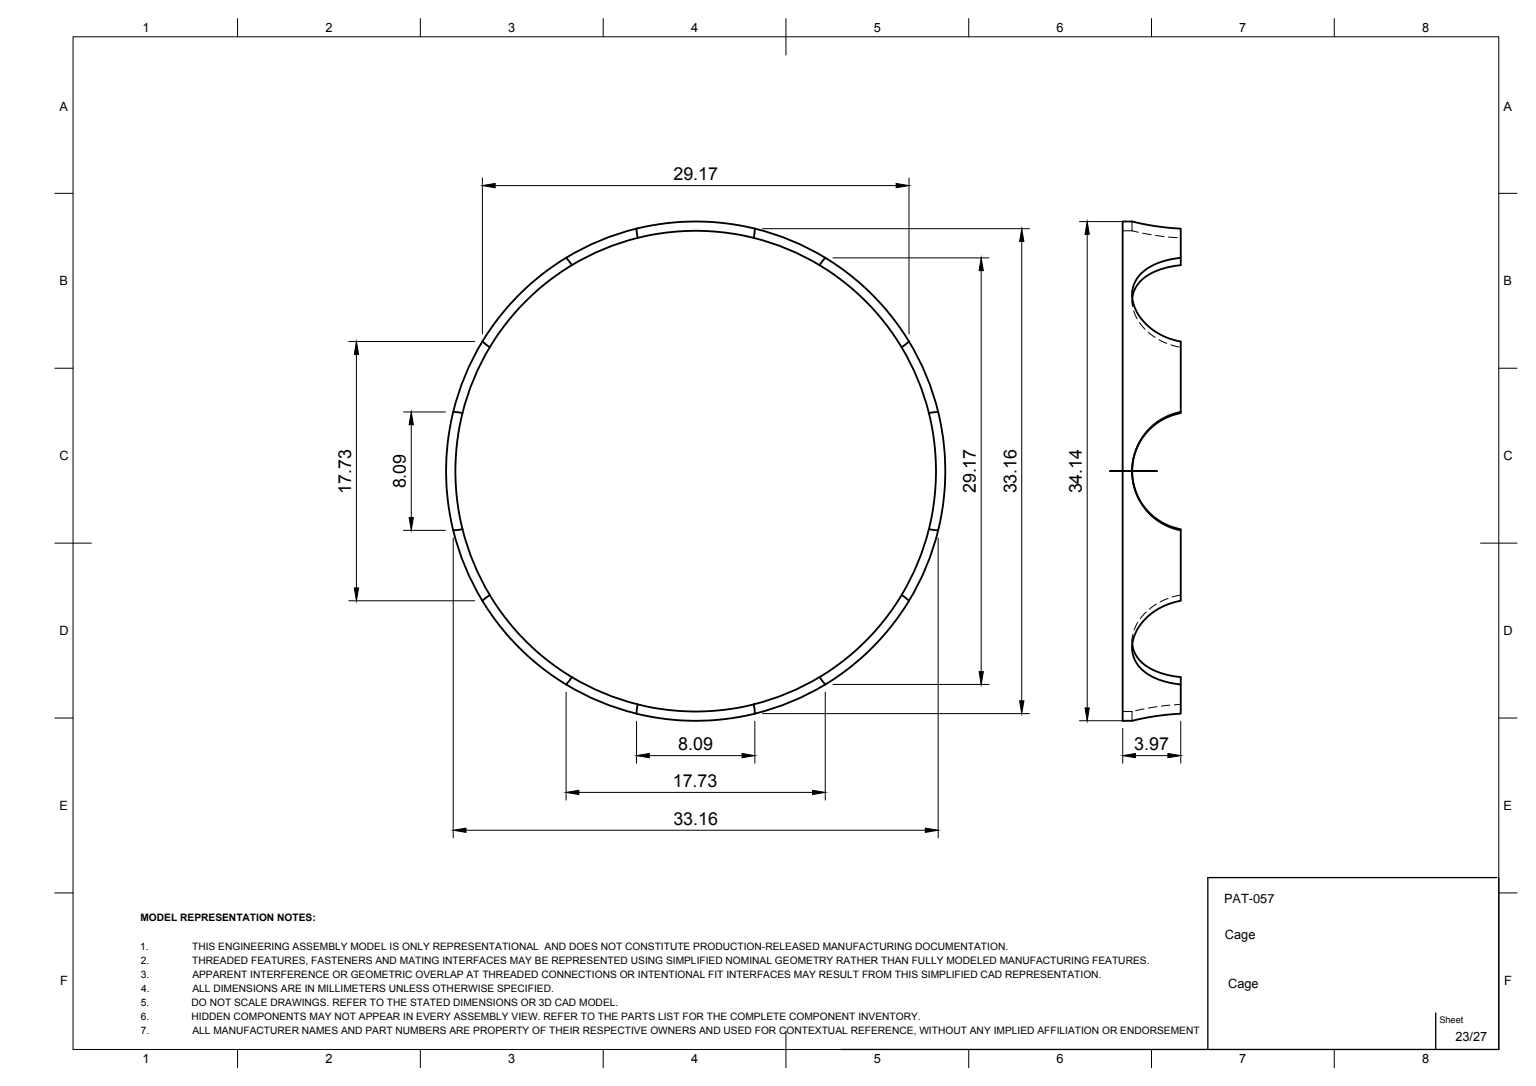
ISO-10303-21;
HEADER;
/* Generated by software containing ST-Developer
 * from STEP Tools, Inc. (www.steptools.com) 
 */

FILE_DESCRIPTION(
/* description */ ('Bearing-mounted hook block'),
/* implementation_level */ '2;1');

FILE_NAME(
/* name */ 'Cage.step',
/* time_stamp */ '2026-10-28T22:30:11-07:00',
/* author */ (''),
/* organization */ (''),
/* preprocessor_version */ 'ST-DEVELOPER v20.2',
/* originating_system */ 'Autodesk Translation Framework v15.17.0.0',
/* authorisation */ '');

FILE_SCHEMA (('AUTOMOTIVE_DESIGN { 1 0 10303 214 3 1 1 }'));
ENDSEC;

DATA;
#10=MECHANICAL_DESIGN_GEOMETRIC_PRESENTATION_REPRESENTATION('',(#347),#7609);
#11=B_SPLINE_CURVE_WITH_KNOTS('',3,(#6806,#6807,#6808,#6809,#6810,#6811,
#6812,#6813,#6814,#6815,#6816,#6817,#6818,#6819,#6820,#6821,#6822,#6823,
#6824,#6825,#6826,#6827),.UNSPECIFIED.,.F.,.F.,(4,2,2,2,2,2,2,2,2,2,4),
(0.0789094028588958,0.210573405340968,0.315860108011452,0.421146810681936,
0.522142632548711,0.623138454415485,0.72413427628226,0.825130098149035,
0.930416800819519,1.03570350349,1.16736750597208),.UNSPECIFIED.);
#12=B_SPLINE_CURVE_WITH_KNOTS('',3,(#6831,#6832,#6833,#6834,#6835,#6836,
#6837,#6838,#6839,#6840,#6841,#6842,#6843,#6844,#6845,#6846,#6847,#6848,
#6849,#6850,#6851,#6852),.UNSPECIFIED.,.F.,.F.,(4,2,2,2,2,2,2,2,2,2,4),
(0.0774793363974613,0.142088896491891,0.284177792983782,0.411119756996526,
0.514392970548519,0.617666184100513,0.720939397652506,0.8242126112045,0.951154575217244,
1.09324347170913,1.15785303180356),.UNSPECIFIED.);
#13=B_SPLINE_CURVE_WITH_KNOTS('',3,(#6858,#6859,#6860,#6861,#6862,#6863,
#6864,#6865,#6866,#6867,#6868,#6869,#6870,#6871,#6872,#6873,#6874,#6875,
#6876,#6877,#6878,#6879),.UNSPECIFIED.,.F.,.F.,(4,2,2,2,2,2,2,2,2,2,4),
(0.0774793363974613,0.142088896491891,0.284177792983782,0.411119756996525,
0.514392970548519,0.617666184100513,0.720939397652506,0.8242126112045,0.951154575217243,
1.09324347170913,1.15785303180356),.UNSPECIFIED.);
#14=B_SPLINE_CURVE_WITH_KNOTS('',3,(#6883,#6884,#6885,#6886,#6887,#6888,
#6889,#6890,#6891,#6892,#6893,#6894,#6895,#6896,#6897,#6898,#6899,#6900,
#6901,#6902,#6903,#6904),.UNSPECIFIED.,.F.,.F.,(4,2,2,2,2,2,2,2,2,2,4),
(0.0774793363974614,0.142088896491891,0.284177792983781,0.411119756996525,
0.514392970548519,0.617666184100512,0.720939397652506,0.824212611204499,
0.951154575217243,1.09324347170913,1.15785303180356),.UNSPECIFIED.);
#15=B_SPLINE_CURVE_WITH_KNOTS('',3,(#6908,#6909,#6910,#6911,#6912,#6913,
#6914,#6915,#6916,#6917,#6918,#6919),.UNSPECIFIED.,.F.,.F.,(4,2,2,2,2,4),
(0.0774793363974613,0.142088896491891,0.284177792983781,0.411119756996525,
0.514392970548519,0.617666184100512),.UNSPECIFIED.);
#16=B_SPLINE_CURVE_WITH_KNOTS('',3,(#6924,#6925,#6926,#6927,#6928,#6929,
#6930,#6931,#6932,#6933,#6934,#6935),.UNSPECIFIED.,.F.,.F.,(4,2,2,2,2,4),
(0.617666184100512,0.720939397652506,0.824212611204499,0.951154575217243,
1.09324347170913,1.15785303180356),.UNSPECIFIED.);
#17=B_SPLINE_CURVE_WITH_KNOTS('',3,(#6939,#6940,#6941,#6942,#6943,#6944,
#6945,#6946,#6947,#6948,#6949,#6950,#6951,#6952,#6953,#6954,#6955,#6956,
#6957,#6958,#6959,#6960),.UNSPECIFIED.,.F.,.F.,(4,2,2,2,2,2,2,2,2,2,4),
(0.0774793363974613,0.142088896491891,0.284177792983782,0.411119756996526,
0.514392970548519,0.617666184100513,0.720939397652507,0.8242126112045,0.951154575217245,
1.09324347170914,1.15785303180356),.UNSPECIFIED.);
#18=B_SPLINE_CURVE_WITH_KNOTS('',3,(#6964,#6965,#6966,#6967,#6968,#6969,
#6970,#6971,#6972,#6973,#6974,#6975,#6976,#6977,#6978,#6979,#6980,#6981,
#6982,#6983,#6984,#6985),.UNSPECIFIED.,.F.,.F.,(4,2,2,2,2,2,2,2,2,2,4),
(0.0774793363974613,0.142088896491891,0.284177792983782,0.411119756996526,
0.514392970548519,0.617666184100513,0.720939397652506,0.824212611204499,
0.951154575217243,1.09324347170913,1.15785303180356),.UNSPECIFIED.);
#19=B_SPLINE_CURVE_WITH_KNOTS('',3,(#6989,#6990,#6991,#6992,#6993,#6994,
#6995,#6996,#6997,#6998,#6999,#7000,#7001,#7002,#7003,#7004,#7005,#7006,
#7007,#7008,#7009,#7010),.UNSPECIFIED.,.F.,.F.,(4,2,2,2,2,2,2,2,2,2,4),
(0.0774793363974613,0.142088896491891,0.284177792983782,0.411119756996526,
0.514392970548519,0.617666184100513,0.720939397652506,0.8242126112045,0.951154575217244,
1.09324347170913,1.15785303180356),.UNSPECIFIED.);
#20=B_SPLINE_CURVE_WITH_KNOTS('',3,(#7014,#7015,#7016,#7017,#7018,#7019,
#7020,#7021,#7022,#7023,#7024,#7025,#7026,#7027,#7028,#7029,#7030,#7031,
#7032,#7033,#7034,#7035),.UNSPECIFIED.,.F.,.F.,(4,2,2,2,2,2,2,2,2,2,4),
(0.0774793363974613,0.142088896491891,0.284177792983782,0.411119756996526,
0.514392970548519,0.617666184100513,0.720939397652506,0.8242126112045,0.951154575217243,
1.09324347170913,1.15785303180356),.UNSPECIFIED.);
#21=B_SPLINE_CURVE_WITH_KNOTS('',3,(#7043,#7044,#7045,#7046,#7047,#7048,
#7049,#7050,#7051,#7052,#7053,#7054,#7055,#7056,#7057,#7058,#7059,#7060,
#7061,#7062,#7063,#7064),.UNSPECIFIED.,.F.,.F.,(4,2,2,2,2,2,2,2,2,2,4),
(0.0789094028588958,0.210573405340968,0.315860108011452,0.421146810681936,
0.522142632548711,0.623138454415485,0.72413427628226,0.825130098149035,
0.930416800819519,1.03570350349,1.16736750597208),.UNSPECIFIED.);
#22=B_SPLINE_CURVE_WITH_KNOTS('',3,(#7072,#7073,#7074,#7075,#7076,#7077,
#7078,#7079,#7080,#7081,#7082,#7083,#7084,#7085,#7086,#7087,#7088,#7089,
#7090,#7091,#7092,#7093),.UNSPECIFIED.,.F.,.F.,(4,2,2,2,2,2,2,2,2,2,4),
(0.0789094028588958,0.210573405340969,0.315860108011453,0.421146810681937,
0.522142632548712,0.623138454415486,0.724134276282261,0.825130098149035,
0.930416800819519,1.03570350349,1.16736750597208),.UNSPECIFIED.);
#23=B_SPLINE_CURVE_WITH_KNOTS('',3,(#7102,#7103,#7104,#7105,#7106,#7107,
#7108,#7109,#7110,#7111,#7112,#7113),.UNSPECIFIED.,.F.,.F.,(4,2,2,2,2,4),
(0.0789094028588958,0.210573405340968,0.315860108011452,0.421146810681937,
0.522142632548711,0.623138454415486),.UNSPECIFIED.);
#24=B_SPLINE_CURVE_WITH_KNOTS('',3,(#7115,#7116,#7117,#7118,#7119,#7120,
#7121,#7122,#7123,#7124,#7125,#7126),.UNSPECIFIED.,.F.,.F.,(4,2,2,2,2,4),
(0.623138454415486,0.72413427628226,0.825130098149035,0.930416800819519,
1.03570350349,1.16736750597208),.UNSPECIFIED.);
#25=B_SPLINE_CURVE_WITH_KNOTS('',3,(#7133,#7134,#7135,#7136,#7137,#7138,
#7139,#7140,#7141,#7142,#7143,#7144,#7145,#7146,#7147,#7148,#7149,#7150,
#7151,#7152,#7153,#7154),.UNSPECIFIED.,.F.,.F.,(4,2,2,2,2,2,2,2,2,2,4),
(0.0789094028588958,0.210573405340968,0.315860108011452,0.421146810681936,
0.522142632548711,0.623138454415486,0.72413427628226,0.825130098149035,
0.930416800819519,1.03570350349,1.16736750597208),.UNSPECIFIED.);
#26=B_SPLINE_CURVE_WITH_KNOTS('',3,(#7162,#7163,#7164,#7165,#7166,#7167,
#7168,#7169,#7170,#7171,#7172,#7173,#7174,#7175,#7176,#7177,#7178,#7179,
#7180,#7181,#7182,#7183),.UNSPECIFIED.,.F.,.F.,(4,2,2,2,2,2,2,2,2,2,4),
(0.0789094028588957,0.210573405340968,0.315860108011452,0.421146810681936,
0.522142632548711,0.623138454415485,0.72413427628226,0.825130098149035,
0.930416800819519,1.03570350349,1.16736750597207),.UNSPECIFIED.);
#27=B_SPLINE_CURVE_WITH_KNOTS('',3,(#7191,#7192,#7193,#7194,#7195,#7196,
#7197,#7198,#7199,#7200,#7201,#7202,#7203,#7204,#7205,#7206,#7207,#7208,
#7209,#7210,#7211,#7212),.UNSPECIFIED.,.F.,.F.,(4,2,2,2,2,2,2,2,2,2,4),
(0.0789094028588958,0.210573405340968,0.315860108011452,0.421146810681936,
0.522142632548711,0.623138454415486,0.72413427628226,0.825130098149035,
0.930416800819519,1.03570350349,1.16736750597208),.UNSPECIFIED.);
#28=B_SPLINE_CURVE_WITH_KNOTS('',3,(#7221,#7222,#7223,#7224,#7225,#7226,
#7227,#7228,#7229,#7230,#7231,#7232,#7233,#7234,#7235,#7236,#7237,#7238,
#7239,#7240,#7241,#7242),.UNSPECIFIED.,.F.,.F.,(4,2,2,2,2,2,2,2,2,2,4),
(0.0789094028588958,0.210573405340968,0.315860108011452,0.421146810681936,
0.522142632548711,0.623138454415485,0.72413427628226,0.825130098149035,
0.930416800819519,1.03570350349,1.16736750597208),.UNSPECIFIED.);
#37=SPHERICAL_SURFACE('',#4562,0.412776);
#38=SPHERICAL_SURFACE('',#4578,0.412776);
#39=SPHERICAL_SURFACE('',#4583,0.412776);
#40=SPHERICAL_SURFACE('',#4588,0.412776);
#41=SPHERICAL_SURFACE('',#4593,0.412776);
#42=SPHERICAL_SURFACE('',#4598,0.412776);
#43=SPHERICAL_SURFACE('',#4603,0.412776);
#44=SPHERICAL_SURFACE('',#4611,0.412776);
#292=SHAPE_REPRESENTATION_RELATIONSHIP('SRR','None',#7741,#316);
#316=ADVANCED_BREP_SHAPE_REPRESENTATION('',(#377),#7601);
#347=STYLED_ITEM('',(#7931),#377);
#377=MANIFOLD_SOLID_BREP('Continuous crown cage',#3945);
#535=LINE('',#6921,#765);
#536=LINE('',#7217,#766);
#765=VECTOR('',#5608,1.706752);
#766=VECTOR('',#5685,1.643248);
#898=CYLINDRICAL_SURFACE('',#4565,1.706752);
#899=CYLINDRICAL_SURFACE('',#4605,1.643248);
#978=FACE_BOUND('',#1466,.T.);
#1155=FACE_OUTER_BOUND('',#1448,.T.);
#1156=FACE_OUTER_BOUND('',#1449,.T.);
#1157=FACE_OUTER_BOUND('',#1450,.T.);
#1158=FACE_OUTER_BOUND('',#1451,.T.);
#1159=FACE_OUTER_BOUND('',#1452,.T.);
#1160=FACE_OUTER_BOUND('',#1453,.T.);
#1161=FACE_OUTER_BOUND('',#1454,.T.);
#1162=FACE_OUTER_BOUND('',#1455,.T.);
#1163=FACE_OUTER_BOUND('',#1456,.T.);
#1164=FACE_OUTER_BOUND('',#1457,.T.);
#1165=FACE_OUTER_BOUND('',#1458,.T.);
#1166=FACE_OUTER_BOUND('',#1459,.T.);
#1167=FACE_OUTER_BOUND('',#1460,.T.);
#1168=FACE_OUTER_BOUND('',#1461,.T.);
#1169=FACE_OUTER_BOUND('',#1462,.T.);
#1170=FACE_OUTER_BOUND('',#1463,.T.);
#1171=FACE_OUTER_BOUND('',#1464,.T.);
#1172=FACE_OUTER_BOUND('',#1465,.T.);
#1173=FACE_OUTER_BOUND('',#1467,.T.);
#1448=EDGE_LOOP('',(#3204,#3205,#3206,#3207));
#1449=EDGE_LOOP('',(#3208,#3209,#3210,#3211,#3212,#3213,#3214,#3215,#3216,
#3217,#3218,#3219,#3220,#3221,#3222,#3223,#3224,#3225,#3226,#3227));
#1450=EDGE_LOOP('',(#3228,#3229,#3230,#3231));
#1451=EDGE_LOOP('',(#3232,#3233,#3234,#3235));
#1452=EDGE_LOOP('',(#3236,#3237,#3238,#3239));
#1453=EDGE_LOOP('',(#3240,#3241,#3242,#3243));
#1454=EDGE_LOOP('',(#3244,#3245,#3246,#3247));
#1455=EDGE_LOOP('',(#3248,#3249,#3250,#3251,#3252,#3253));
#1456=EDGE_LOOP('',(#3254,#3255,#3256,#3257));
#1457=EDGE_LOOP('',(#3258,#3259,#3260,#3261));
#1458=EDGE_LOOP('',(#3262,#3263,#3264,#3265));
#1459=EDGE_LOOP('',(#3266,#3267,#3268,#3269));
#1460=EDGE_LOOP('',(#3270,#3271,#3272,#3273));
#1461=EDGE_LOOP('',(#3274,#3275,#3276,#3277));
#1462=EDGE_LOOP('',(#3278,#3279,#3280,#3281,#3282,#3283,#3284,#3285,#3286,
#3287,#3288,#3289,#3290,#3291,#3292,#3293,#3294,#3295,#3296,#3297));
#1463=EDGE_LOOP('',(#3298,#3299,#3300,#3301));
#1464=EDGE_LOOP('',(#3302,#3303,#3304,#3305));
#1465=EDGE_LOOP('',(#3306));
#1466=EDGE_LOOP('',(#3307));
#1467=EDGE_LOOP('',(#3308,#3309,#3310,#3311));
#1697=CIRCLE('',#4563,0.405071403305639);
#1698=CIRCLE('',#4564,0.405071403305639);
#1699=CIRCLE('',#4566,1.706752);
#1700=CIRCLE('',#4567,1.706752);
#1701=CIRCLE('',#4568,1.706752);
#1702=CIRCLE('',#4569,1.706752);
#1703=CIRCLE('',#4570,1.706752);
#1704=CIRCLE('',#4571,1.706752);
#1705=CIRCLE('',#4572,1.706752);
#1706=CIRCLE('',#4573,1.706752);
#1707=CIRCLE('',#4574,1.706752);
#1708=CIRCLE('',#4576,1.643248);
#1709=CIRCLE('',#4577,0.405071403305639);
#1710=CIRCLE('',#4579,0.405071403305639);
#1711=CIRCLE('',#4581,1.643248);
#1712=CIRCLE('',#4582,0.405071403305639);
#1713=CIRCLE('',#4584,0.405071403305639);
#1714=CIRCLE('',#4586,1.643248);
#1715=CIRCLE('',#4587,0.405071403305639);
#1716=CIRCLE('',#4589,0.405071403305639);
#1717=CIRCLE('',#4591,1.643248);
#1718=CIRCLE('',#4592,0.405071403305639);
#1719=CIRCLE('',#4594,0.405071403305639);
#1720=CIRCLE('',#4596,1.643248);
#1721=CIRCLE('',#4597,0.405071403305639);
#1722=CIRCLE('',#4599,0.405071403305639);
#1723=CIRCLE('',#4601,1.643248);
#1724=CIRCLE('',#4602,0.405071403305639);
#1725=CIRCLE('',#4604,0.405071403305639);
#1726=CIRCLE('',#4606,1.643248);
#1727=CIRCLE('',#4607,1.643248);
#1728=CIRCLE('',#4608,1.643248);
#1729=CIRCLE('',#4610,0.405071403305639);
#1730=CIRCLE('',#4612,0.405071403305639);
#1988=VERTEX_POINT('',#6804);
#1989=VERTEX_POINT('',#6805);
#1990=VERTEX_POINT('',#6828);
#1991=VERTEX_POINT('',#6830);
#1992=VERTEX_POINT('',#6855);
#1993=VERTEX_POINT('',#6857);
#1994=VERTEX_POINT('',#6880);
#1995=VERTEX_POINT('',#6882);
#1996=VERTEX_POINT('',#6905);
#1997=VERTEX_POINT('',#6907);
#1998=VERTEX_POINT('',#6920);
#1999=VERTEX_POINT('',#6923);
#2000=VERTEX_POINT('',#6936);
#2001=VERTEX_POINT('',#6938);
#2002=VERTEX_POINT('',#6961);
#2003=VERTEX_POINT('',#6963);
#2004=VERTEX_POINT('',#6986);
#2005=VERTEX_POINT('',#6988);
#2006=VERTEX_POINT('',#7011);
#2007=VERTEX_POINT('',#7013);
#2008=VERTEX_POINT('',#7038);
#2009=VERTEX_POINT('',#7042);
#2010=VERTEX_POINT('',#7067);
#2011=VERTEX_POINT('',#7071);
#2012=VERTEX_POINT('',#7096);
#2013=VERTEX_POINT('',#7100);
#2014=VERTEX_POINT('',#7101);
#2015=VERTEX_POINT('',#7128);
#2016=VERTEX_POINT('',#7132);
#2017=VERTEX_POINT('',#7157);
#2018=VERTEX_POINT('',#7161);
#2019=VERTEX_POINT('',#7186);
#2020=VERTEX_POINT('',#7190);
#2021=VERTEX_POINT('',#7215);
#2022=VERTEX_POINT('',#7218);
#2023=VERTEX_POINT('',#7220);
#2412=EDGE_CURVE('',#1988,#1989,#11,.T.);
#2413=EDGE_CURVE('',#1990,#1988,#1697,.T.);
#2414=EDGE_CURVE('',#1991,#1990,#12,.T.);
#2415=EDGE_CURVE('',#1989,#1991,#1698,.T.);
#2416=EDGE_CURVE('',#1992,#1990,#1699,.T.);
#2417=EDGE_CURVE('',#1992,#1993,#13,.T.);
#2418=EDGE_CURVE('',#1994,#1993,#1700,.T.);
#2419=EDGE_CURVE('',#1994,#1995,#14,.T.);
#2420=EDGE_CURVE('',#1996,#1995,#1701,.T.);
#2421=EDGE_CURVE('',#1996,#1997,#15,.T.);
#2422=EDGE_CURVE('',#1997,#1998,#535,.T.);
#2423=EDGE_CURVE('',#1998,#1998,#1702,.T.);
#2424=EDGE_CURVE('',#1997,#1999,#16,.T.);
#2425=EDGE_CURVE('',#2000,#1999,#1703,.T.);
#2426=EDGE_CURVE('',#2000,#2001,#17,.T.);
#2427=EDGE_CURVE('',#2002,#2001,#1704,.T.);
#2428=EDGE_CURVE('',#2002,#2003,#18,.T.);
#2429=EDGE_CURVE('',#2004,#2003,#1705,.T.);
#2430=EDGE_CURVE('',#2004,#2005,#19,.T.);
#2431=EDGE_CURVE('',#2006,#2005,#1706,.T.);
#2432=EDGE_CURVE('',#2006,#2007,#20,.T.);
#2433=EDGE_CURVE('',#1991,#2007,#1707,.T.);
#2434=EDGE_CURVE('',#1988,#2008,#1708,.T.);
#2435=EDGE_CURVE('',#2008,#1992,#1709,.T.);
#2436=EDGE_CURVE('',#2009,#2008,#21,.T.);
#2437=EDGE_CURVE('',#1993,#2009,#1710,.T.);
#2438=EDGE_CURVE('',#2009,#2010,#1711,.T.);
#2439=EDGE_CURVE('',#2010,#1994,#1712,.T.);
#2440=EDGE_CURVE('',#2011,#2010,#22,.T.);
#2441=EDGE_CURVE('',#1995,#2011,#1713,.T.);
#2442=EDGE_CURVE('',#2011,#2012,#1714,.T.);
#2443=EDGE_CURVE('',#2012,#1996,#1715,.T.);
#2444=EDGE_CURVE('',#2013,#2014,#23,.T.);
#2445=EDGE_CURVE('',#1999,#2013,#1716,.T.);
#2446=EDGE_CURVE('',#2014,#2012,#24,.T.);
#2447=EDGE_CURVE('',#2013,#2015,#1717,.T.);
#2448=EDGE_CURVE('',#2015,#2000,#1718,.T.);
#2449=EDGE_CURVE('',#2016,#2015,#25,.T.);
#2450=EDGE_CURVE('',#2001,#2016,#1719,.T.);
#2451=EDGE_CURVE('',#2016,#2017,#1720,.T.);
#2452=EDGE_CURVE('',#2017,#2002,#1721,.T.);
#2453=EDGE_CURVE('',#2018,#2017,#26,.T.);
#2454=EDGE_CURVE('',#2003,#2018,#1722,.T.);
#2455=EDGE_CURVE('',#2018,#2019,#1723,.T.);
#2456=EDGE_CURVE('',#2019,#2004,#1724,.T.);
#2457=EDGE_CURVE('',#2020,#2019,#27,.T.);
#2458=EDGE_CURVE('',#2005,#2020,#1725,.T.);
#2459=EDGE_CURVE('',#2021,#2021,#1726,.T.);
#2460=EDGE_CURVE('',#2021,#2014,#536,.T.);
#2461=EDGE_CURVE('',#2022,#1989,#1727,.T.);
#2462=EDGE_CURVE('',#2022,#2023,#28,.T.);
#2463=EDGE_CURVE('',#2020,#2023,#1728,.T.);
#2464=EDGE_CURVE('',#2007,#2022,#1729,.T.);
#2465=EDGE_CURVE('',#2023,#2006,#1730,.T.);
#3204=ORIENTED_EDGE('',*,*,#2412,.F.);
#3205=ORIENTED_EDGE('',*,*,#2413,.F.);
#3206=ORIENTED_EDGE('',*,*,#2414,.F.);
#3207=ORIENTED_EDGE('',*,*,#2415,.F.);
#3208=ORIENTED_EDGE('',*,*,#2414,.T.);
#3209=ORIENTED_EDGE('',*,*,#2416,.F.);
#3210=ORIENTED_EDGE('',*,*,#2417,.T.);
#3211=ORIENTED_EDGE('',*,*,#2418,.F.);
#3212=ORIENTED_EDGE('',*,*,#2419,.T.);
#3213=ORIENTED_EDGE('',*,*,#2420,.F.);
#3214=ORIENTED_EDGE('',*,*,#2421,.T.);
#3215=ORIENTED_EDGE('',*,*,#2422,.T.);
#3216=ORIENTED_EDGE('',*,*,#2423,.F.);
#3217=ORIENTED_EDGE('',*,*,#2422,.F.);
#3218=ORIENTED_EDGE('',*,*,#2424,.T.);
#3219=ORIENTED_EDGE('',*,*,#2425,.F.);
#3220=ORIENTED_EDGE('',*,*,#2426,.T.);
#3221=ORIENTED_EDGE('',*,*,#2427,.F.);
#3222=ORIENTED_EDGE('',*,*,#2428,.T.);
#3223=ORIENTED_EDGE('',*,*,#2429,.F.);
#3224=ORIENTED_EDGE('',*,*,#2430,.T.);
#3225=ORIENTED_EDGE('',*,*,#2431,.F.);
#3226=ORIENTED_EDGE('',*,*,#2432,.T.);
#3227=ORIENTED_EDGE('',*,*,#2433,.F.);
#3228=ORIENTED_EDGE('',*,*,#2413,.T.);
#3229=ORIENTED_EDGE('',*,*,#2434,.T.);
#3230=ORIENTED_EDGE('',*,*,#2435,.T.);
#3231=ORIENTED_EDGE('',*,*,#2416,.T.);
#3232=ORIENTED_EDGE('',*,*,#2436,.F.);
#3233=ORIENTED_EDGE('',*,*,#2437,.F.);
#3234=ORIENTED_EDGE('',*,*,#2417,.F.);
#3235=ORIENTED_EDGE('',*,*,#2435,.F.);
#3236=ORIENTED_EDGE('',*,*,#2437,.T.);
#3237=ORIENTED_EDGE('',*,*,#2438,.T.);
#3238=ORIENTED_EDGE('',*,*,#2439,.T.);
#3239=ORIENTED_EDGE('',*,*,#2418,.T.);
#3240=ORIENTED_EDGE('',*,*,#2440,.F.);
#3241=ORIENTED_EDGE('',*,*,#2441,.F.);
#3242=ORIENTED_EDGE('',*,*,#2419,.F.);
#3243=ORIENTED_EDGE('',*,*,#2439,.F.);
#3244=ORIENTED_EDGE('',*,*,#2441,.T.);
#3245=ORIENTED_EDGE('',*,*,#2442,.T.);
#3246=ORIENTED_EDGE('',*,*,#2443,.T.);
#3247=ORIENTED_EDGE('',*,*,#2420,.T.);
#3248=ORIENTED_EDGE('',*,*,#2444,.F.);
#3249=ORIENTED_EDGE('',*,*,#2445,.F.);
#3250=ORIENTED_EDGE('',*,*,#2424,.F.);
#3251=ORIENTED_EDGE('',*,*,#2421,.F.);
#3252=ORIENTED_EDGE('',*,*,#2443,.F.);
#3253=ORIENTED_EDGE('',*,*,#2446,.F.);
#3254=ORIENTED_EDGE('',*,*,#2445,.T.);
#3255=ORIENTED_EDGE('',*,*,#2447,.T.);
#3256=ORIENTED_EDGE('',*,*,#2448,.T.);
#3257=ORIENTED_EDGE('',*,*,#2425,.T.);
#3258=ORIENTED_EDGE('',*,*,#2449,.F.);
#3259=ORIENTED_EDGE('',*,*,#2450,.F.);
#3260=ORIENTED_EDGE('',*,*,#2426,.F.);
#3261=ORIENTED_EDGE('',*,*,#2448,.F.);
#3262=ORIENTED_EDGE('',*,*,#2450,.T.);
#3263=ORIENTED_EDGE('',*,*,#2451,.T.);
#3264=ORIENTED_EDGE('',*,*,#2452,.T.);
#3265=ORIENTED_EDGE('',*,*,#2427,.T.);
#3266=ORIENTED_EDGE('',*,*,#2453,.F.);
#3267=ORIENTED_EDGE('',*,*,#2454,.F.);
#3268=ORIENTED_EDGE('',*,*,#2428,.F.);
#3269=ORIENTED_EDGE('',*,*,#2452,.F.);
#3270=ORIENTED_EDGE('',*,*,#2454,.T.);
#3271=ORIENTED_EDGE('',*,*,#2455,.T.);
#3272=ORIENTED_EDGE('',*,*,#2456,.T.);
#3273=ORIENTED_EDGE('',*,*,#2429,.T.);
#3274=ORIENTED_EDGE('',*,*,#2430,.F.);
#3275=ORIENTED_EDGE('',*,*,#2456,.F.);
#3276=ORIENTED_EDGE('',*,*,#2457,.F.);
#3277=ORIENTED_EDGE('',*,*,#2458,.F.);
#3278=ORIENTED_EDGE('',*,*,#2459,.F.);
#3279=ORIENTED_EDGE('',*,*,#2460,.T.);
#3280=ORIENTED_EDGE('',*,*,#2446,.T.);
#3281=ORIENTED_EDGE('',*,*,#2442,.F.);
#3282=ORIENTED_EDGE('',*,*,#2440,.T.);
#3283=ORIENTED_EDGE('',*,*,#2438,.F.);
#3284=ORIENTED_EDGE('',*,*,#2436,.T.);
#3285=ORIENTED_EDGE('',*,*,#2434,.F.);
#3286=ORIENTED_EDGE('',*,*,#2412,.T.);
#3287=ORIENTED_EDGE('',*,*,#2461,.F.);
#3288=ORIENTED_EDGE('',*,*,#2462,.T.);
#3289=ORIENTED_EDGE('',*,*,#2463,.F.);
#3290=ORIENTED_EDGE('',*,*,#2457,.T.);
#3291=ORIENTED_EDGE('',*,*,#2455,.F.);
#3292=ORIENTED_EDGE('',*,*,#2453,.T.);
#3293=ORIENTED_EDGE('',*,*,#2451,.F.);
#3294=ORIENTED_EDGE('',*,*,#2449,.T.);
#3295=ORIENTED_EDGE('',*,*,#2447,.F.);
#3296=ORIENTED_EDGE('',*,*,#2444,.T.);
#3297=ORIENTED_EDGE('',*,*,#2460,.F.);
#3298=ORIENTED_EDGE('',*,*,#2415,.T.);
#3299=ORIENTED_EDGE('',*,*,#2433,.T.);
#3300=ORIENTED_EDGE('',*,*,#2464,.T.);
#3301=ORIENTED_EDGE('',*,*,#2461,.T.);
#3302=ORIENTED_EDGE('',*,*,#2432,.F.);
#3303=ORIENTED_EDGE('',*,*,#2465,.F.);
#3304=ORIENTED_EDGE('',*,*,#2462,.F.);
#3305=ORIENTED_EDGE('',*,*,#2464,.F.);
#3306=ORIENTED_EDGE('',*,*,#2423,.T.);
#3307=ORIENTED_EDGE('',*,*,#2459,.T.);
#3308=ORIENTED_EDGE('',*,*,#2458,.T.);
#3309=ORIENTED_EDGE('',*,*,#2463,.T.);
#3310=ORIENTED_EDGE('',*,*,#2465,.T.);
#3311=ORIENTED_EDGE('',*,*,#2431,.T.);
#3635=PLANE('',#4575);
#3636=PLANE('',#4580);
#3637=PLANE('',#4585);
#3638=PLANE('',#4590);
#3639=PLANE('',#4595);
#3640=PLANE('',#4600);
#3641=PLANE('',#4609);
#3642=PLANE('',#4613);
#3643=PLANE('',#4614);
#3837=ADVANCED_FACE('',(#1155),#37,.F.);
#3838=ADVANCED_FACE('',(#1156),#898,.T.);
#3839=ADVANCED_FACE('',(#1157),#3635,.T.);
#3840=ADVANCED_FACE('',(#1158),#38,.F.);
#3841=ADVANCED_FACE('',(#1159),#3636,.T.);
#3842=ADVANCED_FACE('',(#1160),#39,.F.);
#3843=ADVANCED_FACE('',(#1161),#3637,.T.);
#3844=ADVANCED_FACE('',(#1162),#40,.F.);
#3845=ADVANCED_FACE('',(#1163),#3638,.T.);
#3846=ADVANCED_FACE('',(#1164),#41,.F.);
#3847=ADVANCED_FACE('',(#1165),#3639,.T.);
#3848=ADVANCED_FACE('',(#1166),#42,.F.);
#3849=ADVANCED_FACE('',(#1167),#3640,.T.);
#3850=ADVANCED_FACE('',(#1168),#43,.F.);
#3851=ADVANCED_FACE('',(#1169),#899,.F.);
#3852=ADVANCED_FACE('',(#1170),#3641,.T.);
#3853=ADVANCED_FACE('',(#1171),#44,.F.);
#3854=ADVANCED_FACE('',(#1172,#978),#3642,.T.);
#3855=ADVANCED_FACE('',(#1173),#3643,.T.);
#3945=CLOSED_SHELL('',(#3837,#3838,#3839,#3840,#3841,#3842,#3843,#3844,
#3845,#3846,#3847,#3848,#3849,#3850,#3851,#3852,#3853,#3854,#3855));
#4561=AXIS2_PLACEMENT_3D('',#6802,#5592,#5593);
#4562=AXIS2_PLACEMENT_3D('',#6803,#5594,#5595);
#4563=AXIS2_PLACEMENT_3D('',#6829,#5596,#5597);
#4564=AXIS2_PLACEMENT_3D('',#6853,#5598,#5599);
#4565=AXIS2_PLACEMENT_3D('',#6854,#5600,#5601);
#4566=AXIS2_PLACEMENT_3D('',#6856,#5602,#5603);
#4567=AXIS2_PLACEMENT_3D('',#6881,#5604,#5605);
#4568=AXIS2_PLACEMENT_3D('',#6906,#5606,#5607);
#4569=AXIS2_PLACEMENT_3D('',#6922,#5609,#5610);
#4570=AXIS2_PLACEMENT_3D('',#6937,#5611,#5612);
#4571=AXIS2_PLACEMENT_3D('',#6962,#5613,#5614);
#4572=AXIS2_PLACEMENT_3D('',#6987,#5615,#5616);
#4573=AXIS2_PLACEMENT_3D('',#7012,#5617,#5618);
#4574=AXIS2_PLACEMENT_3D('',#7036,#5619,#5620);
#4575=AXIS2_PLACEMENT_3D('',#7037,#5621,#5622);
#4576=AXIS2_PLACEMENT_3D('',#7039,#5623,#5624);
#4577=AXIS2_PLACEMENT_3D('',#7040,#5625,#5626);
#4578=AXIS2_PLACEMENT_3D('',#7041,#5627,#5628);
#4579=AXIS2_PLACEMENT_3D('',#7065,#5629,#5630);
#4580=AXIS2_PLACEMENT_3D('',#7066,#5631,#5632);
#4581=AXIS2_PLACEMENT_3D('',#7068,#5633,#5634);
#4582=AXIS2_PLACEMENT_3D('',#7069,#5635,#5636);
#4583=AXIS2_PLACEMENT_3D('',#7070,#5637,#5638);
#4584=AXIS2_PLACEMENT_3D('',#7094,#5639,#5640);
#4585=AXIS2_PLACEMENT_3D('',#7095,#5641,#5642);
#4586=AXIS2_PLACEMENT_3D('',#7097,#5643,#5644);
#4587=AXIS2_PLACEMENT_3D('',#7098,#5645,#5646);
#4588=AXIS2_PLACEMENT_3D('',#7099,#5647,#5648);
#4589=AXIS2_PLACEMENT_3D('',#7114,#5649,#5650);
#4590=AXIS2_PLACEMENT_3D('',#7127,#5651,#5652);
#4591=AXIS2_PLACEMENT_3D('',#7129,#5653,#5654);
#4592=AXIS2_PLACEMENT_3D('',#7130,#5655,#5656);
#4593=AXIS2_PLACEMENT_3D('',#7131,#5657,#5658);
#4594=AXIS2_PLACEMENT_3D('',#7155,#5659,#5660);
#4595=AXIS2_PLACEMENT_3D('',#7156,#5661,#5662);
#4596=AXIS2_PLACEMENT_3D('',#7158,#5663,#5664);
#4597=AXIS2_PLACEMENT_3D('',#7159,#5665,#5666);
#4598=AXIS2_PLACEMENT_3D('',#7160,#5667,#5668);
#4599=AXIS2_PLACEMENT_3D('',#7184,#5669,#5670);
#4600=AXIS2_PLACEMENT_3D('',#7185,#5671,#5672);
#4601=AXIS2_PLACEMENT_3D('',#7187,#5673,#5674);
#4602=AXIS2_PLACEMENT_3D('',#7188,#5675,#5676);
#4603=AXIS2_PLACEMENT_3D('',#7189,#5677,#5678);
#4604=AXIS2_PLACEMENT_3D('',#7213,#5679,#5680);
#4605=AXIS2_PLACEMENT_3D('',#7214,#5681,#5682);
#4606=AXIS2_PLACEMENT_3D('',#7216,#5683,#5684);
#4607=AXIS2_PLACEMENT_3D('',#7219,#5686,#5687);
#4608=AXIS2_PLACEMENT_3D('',#7243,#5688,#5689);
#4609=AXIS2_PLACEMENT_3D('',#7244,#5690,#5691);
#4610=AXIS2_PLACEMENT_3D('',#7245,#5692,#5693);
#4611=AXIS2_PLACEMENT_3D('',#7246,#5694,#5695);
#4612=AXIS2_PLACEMENT_3D('',#7247,#5696,#5697);
#4613=AXIS2_PLACEMENT_3D('',#7248,#5698,#5699);
#4614=AXIS2_PLACEMENT_3D('',#7249,#5700,#5701);
#5592=DIRECTION('axis',(0.,0.,1.));
#5593=DIRECTION('refdir',(1.,0.,0.));
#5594=DIRECTION('center_axis',(0.,0.,1.));
#5595=DIRECTION('ref_axis',(1.,0.,0.));
#5596=DIRECTION('center_axis',(0.,-1.,0.));
#5597=DIRECTION('ref_axis',(0.,0.,-1.));
#5598=DIRECTION('center_axis',(0.,-1.,0.));
#5599=DIRECTION('ref_axis',(0.,0.,-1.));
#5600=DIRECTION('center_axis',(0.,1.,0.));
#5601=DIRECTION('ref_axis',(1.,0.,0.));
#5602=DIRECTION('center_axis',(0.,1.,0.));
#5603=DIRECTION('ref_axis',(1.,0.,0.));
#5604=DIRECTION('center_axis',(0.,1.,0.));
#5605=DIRECTION('ref_axis',(1.,0.,0.));
#5606=DIRECTION('center_axis',(0.,1.,0.));
#5607=DIRECTION('ref_axis',(1.,0.,0.));
#5608=DIRECTION('',(0.,-1.,0.));
#5609=DIRECTION('center_axis',(0.,-1.,0.));
#5610=DIRECTION('ref_axis',(1.,0.,0.));
#5611=DIRECTION('center_axis',(0.,1.,0.));
#5612=DIRECTION('ref_axis',(1.,0.,0.));
#5613=DIRECTION('center_axis',(0.,1.,0.));
#5614=DIRECTION('ref_axis',(1.,0.,0.));
#5615=DIRECTION('center_axis',(0.,1.,0.));
#5616=DIRECTION('ref_axis',(1.,0.,0.));
#5617=DIRECTION('center_axis',(0.,1.,0.));
#5618=DIRECTION('ref_axis',(1.,0.,0.));
#5619=DIRECTION('center_axis',(0.,1.,0.));
#5620=DIRECTION('ref_axis',(1.,0.,0.));
#5621=DIRECTION('center_axis',(0.,1.,0.));
#5622=DIRECTION('ref_axis',(1.,0.,0.));
#5623=DIRECTION('center_axis',(0.,-1.,0.));
#5624=DIRECTION('ref_axis',(1.,0.,0.));
#5625=DIRECTION('center_axis',(0.,-1.,0.));
#5626=DIRECTION('ref_axis',(0.,0.,-1.));
#5627=DIRECTION('center_axis',(6.12323399573677E-17,0.,1.));
#5628=DIRECTION('ref_axis',(1.,0.,0.));
#5629=DIRECTION('center_axis',(0.,-1.,0.));
#5630=DIRECTION('ref_axis',(0.,0.,-1.));
#5631=DIRECTION('center_axis',(0.,1.,0.));
#5632=DIRECTION('ref_axis',(1.,0.,0.));
#5633=DIRECTION('center_axis',(0.,-1.,0.));
#5634=DIRECTION('ref_axis',(1.,0.,0.));
#5635=DIRECTION('center_axis',(0.,-1.,0.));
#5636=DIRECTION('ref_axis',(0.,0.,-1.));
#5637=DIRECTION('center_axis',(0.,0.,1.));
#5638=DIRECTION('ref_axis',(1.,0.,0.));
#5639=DIRECTION('center_axis',(0.,-1.,0.));
#5640=DIRECTION('ref_axis',(0.,0.,-1.));
#5641=DIRECTION('center_axis',(0.,1.,0.));
#5642=DIRECTION('ref_axis',(1.,0.,0.));
#5643=DIRECTION('center_axis',(0.,-1.,0.));
#5644=DIRECTION('ref_axis',(1.,0.,0.));
#5645=DIRECTION('center_axis',(0.,-1.,0.));
#5646=DIRECTION('ref_axis',(0.,0.,-1.));
#5647=DIRECTION('center_axis',(0.,0.,1.));
#5648=DIRECTION('ref_axis',(1.,0.,0.));
#5649=DIRECTION('center_axis',(0.,-1.,0.));
#5650=DIRECTION('ref_axis',(0.,0.,-1.));
#5651=DIRECTION('center_axis',(0.,1.,0.));
#5652=DIRECTION('ref_axis',(1.,0.,0.));
#5653=DIRECTION('center_axis',(0.,-1.,0.));
#5654=DIRECTION('ref_axis',(1.,0.,0.));
#5655=DIRECTION('center_axis',(0.,-1.,0.));
#5656=DIRECTION('ref_axis',(0.,0.,-1.));
#5657=DIRECTION('center_axis',(0.,0.,1.));
#5658=DIRECTION('ref_axis',(1.,0.,0.));
#5659=DIRECTION('center_axis',(0.,-1.,0.));
#5660=DIRECTION('ref_axis',(0.,0.,-1.));
#5661=DIRECTION('center_axis',(0.,1.,0.));
#5662=DIRECTION('ref_axis',(1.,0.,0.));
#5663=DIRECTION('center_axis',(0.,-1.,0.));
#5664=DIRECTION('ref_axis',(1.,0.,0.));
#5665=DIRECTION('center_axis',(0.,-1.,0.));
#5666=DIRECTION('ref_axis',(0.,0.,-1.));
#5667=DIRECTION('center_axis',(6.12323399573676E-17,0.,1.));
#5668=DIRECTION('ref_axis',(1.,0.,0.));
#5669=DIRECTION('center_axis',(0.,-1.,0.));
#5670=DIRECTION('ref_axis',(0.,0.,-1.));
#5671=DIRECTION('center_axis',(0.,1.,0.));
#5672=DIRECTION('ref_axis',(1.,0.,0.));
#5673=DIRECTION('center_axis',(0.,-1.,0.));
#5674=DIRECTION('ref_axis',(1.,0.,0.));
#5675=DIRECTION('center_axis',(0.,-1.,0.));
#5676=DIRECTION('ref_axis',(0.,0.,-1.));
#5677=DIRECTION('center_axis',(0.,0.,1.));
#5678=DIRECTION('ref_axis',(1.,0.,0.));
#5679=DIRECTION('center_axis',(0.,-1.,0.));
#5680=DIRECTION('ref_axis',(0.,0.,-1.));
#5681=DIRECTION('center_axis',(0.,1.,0.));
#5682=DIRECTION('ref_axis',(1.,0.,0.));
#5683=DIRECTION('center_axis',(0.,1.,0.));
#5684=DIRECTION('ref_axis',(1.,0.,0.));
#5685=DIRECTION('',(0.,1.,0.));
#5686=DIRECTION('center_axis',(0.,-1.,0.));
#5687=DIRECTION('ref_axis',(1.,0.,0.));
#5688=DIRECTION('center_axis',(0.,-1.,0.));
#5689=DIRECTION('ref_axis',(1.,0.,0.));
#5690=DIRECTION('center_axis',(0.,1.,0.));
#5691=DIRECTION('ref_axis',(1.,0.,0.));
#5692=DIRECTION('center_axis',(0.,-1.,0.));
#5693=DIRECTION('ref_axis',(0.,0.,-1.));
#5694=DIRECTION('center_axis',(0.,0.,1.));
#5695=DIRECTION('ref_axis',(1.,0.,0.));
#5696=DIRECTION('center_axis',(0.,-1.,0.));
#5697=DIRECTION('ref_axis',(0.,0.,-1.));
#5698=DIRECTION('center_axis',(0.,-1.,0.));
#5699=DIRECTION('ref_axis',(-1.,0.,0.));
#5700=DIRECTION('center_axis',(0.,1.,0.));
#5701=DIRECTION('ref_axis',(1.,0.,0.));
#6802=CARTESIAN_POINT('',(0.,0.,0.));
#6803=CARTESIAN_POINT('Origin',(1.18440385848747,0.,1.18440385848747));
#6804=CARTESIAN_POINT('',(0.846804978391753,-0.07938,1.40825612658882));
#6805=CARTESIAN_POINT('',(1.40825612658882,-0.07938,0.846804978391754));
#6806=CARTESIAN_POINT('Ctrl Pts',(0.846804978391752,-0.0793800000000001,
1.40825612658882));
#6807=CARTESIAN_POINT('Ctrl Pts',(0.854205272175554,-0.123401821157026,
1.40380622184538));
#6808=CARTESIAN_POINT('Ctrl Pts',(0.867957148219441,-0.166543350814306,
1.39550172959303));
#6809=CARTESIAN_POINT('Ctrl Pts',(0.902193646979982,-0.237231147975234,
1.3735491215176));
#6810=CARTESIAN_POINT('Ctrl Pts',(0.920778333482564,-0.266264900654909,
1.36127834356734));
#6811=CARTESIAN_POINT('Ctrl Pts',(0.962485392528369,-0.317195968905306,
1.33211611256184));
#6812=CARTESIAN_POINT('Ctrl Pts',(0.985600426557816,-0.33909093068465,1.31521005565926));
#6813=CARTESIAN_POINT('Ctrl Pts',(1.03253285680459,-0.373586846396559,1.27866649102984));
#6814=CARTESIAN_POINT('Ctrl Pts',(1.05871835910697,-0.388086240756494,1.25722555095714));
#6815=CARTESIAN_POINT('Ctrl Pts',(1.11153475808518,-0.407068917407805,1.2107812086231));
#6816=CARTESIAN_POINT('Ctrl Pts',(1.13814686046673,-0.411552957311693,1.18575674747573));
#6817=CARTESIAN_POINT('Ctrl Pts',(1.18575674747573,-0.411552957311693,1.13814686046673));
#6818=CARTESIAN_POINT('Ctrl Pts',(1.2107812086231,-0.407068917407805,1.11153475808518));
#6819=CARTESIAN_POINT('Ctrl Pts',(1.25722555095713,-0.388086240756494,1.05871835910697));
#6820=CARTESIAN_POINT('Ctrl Pts',(1.27866649102984,-0.373586846396559,1.03253285680459));
#6821=CARTESIAN_POINT('Ctrl Pts',(1.31521005565926,-0.33909093068465,0.985600426557816));
#6822=CARTESIAN_POINT('Ctrl Pts',(1.33211611256184,-0.317195968905306,0.962485392528369));
#6823=CARTESIAN_POINT('Ctrl Pts',(1.36127834356734,-0.266264900654909,0.920778333482565));
#6824=CARTESIAN_POINT('Ctrl Pts',(1.3735491215176,-0.237231147975234,0.902193646979983));
#6825=CARTESIAN_POINT('Ctrl Pts',(1.39550172959303,-0.166543350814306,0.867957148219442));
#6826=CARTESIAN_POINT('Ctrl Pts',(1.40380622184538,-0.123401821157026,0.854205272175555));
#6827=CARTESIAN_POINT('Ctrl Pts',(1.40825612658882,-0.0793800000000001,
0.846804978391753));
#6828=CARTESIAN_POINT('',(0.886256117232623,-0.07938,1.45861320581289));
#6829=CARTESIAN_POINT('Origin',(1.18440385848747,-0.07938,1.18440385848747));
#6830=CARTESIAN_POINT('',(1.45861320581289,-0.07938,0.886256117232624));
#6831=CARTESIAN_POINT('Ctrl Pts',(1.45861320581289,-0.0793800000000001,
0.886256117232623));
#6832=CARTESIAN_POINT('Ctrl Pts',(1.45630208793976,-0.101649918886749,0.890059788636852));
#6833=CARTESIAN_POINT('Ctrl Pts',(1.45296717977858,-0.123823518623746,0.895520212222107));
#6834=CARTESIAN_POINT('Ctrl Pts',(1.43904931717599,-0.192480977588836,0.917859913453975));
#6835=CARTESIAN_POINT('Ctrl Pts',(1.4243271592157,-0.236152929235938,0.940896403863072));
#6836=CARTESIAN_POINT('Ctrl Pts',(1.39055359345152,-0.303141259068212,0.990027513266106));
#6837=CARTESIAN_POINT('Ctrl Pts',(1.36743459453896,-0.335108247315849,1.02199477007745));
#6838=CARTESIAN_POINT('Ctrl Pts',(1.32643091652006,-0.373243761060364,1.07446535104584));
#6839=CARTESIAN_POINT('Ctrl Pts',(1.30441816675528,-0.387888272594439,1.10126842659597));
#6840=CARTESIAN_POINT('Ctrl Pts',(1.25681160160691,-0.407041111792943,1.15530234155453));
#6841=CARTESIAN_POINT('Ctrl Pts',(1.23119764287622,-0.411552957311693,1.18251418313119));
#6842=CARTESIAN_POINT('Ctrl Pts',(1.18251418313119,-0.411552957311693,1.23119764287622));
#6843=CARTESIAN_POINT('Ctrl Pts',(1.15530234155453,-0.407041111792943,1.25681160160691));
#6844=CARTESIAN_POINT('Ctrl Pts',(1.10126842659597,-0.387888272594439,1.30441816675528));
#6845=CARTESIAN_POINT('Ctrl Pts',(1.07446535104584,-0.373243761060364,1.32643091652006));
#6846=CARTESIAN_POINT('Ctrl Pts',(1.02199477007745,-0.335108247315848,1.36743459453896));
#6847=CARTESIAN_POINT('Ctrl Pts',(0.990027513266105,-0.303141259068211,
1.39055359345152));
#6848=CARTESIAN_POINT('Ctrl Pts',(0.940896403863071,-0.236152929235937,
1.42432715921571));
#6849=CARTESIAN_POINT('Ctrl Pts',(0.917859913453974,-0.192480977588835,
1.43904931717599));
#6850=CARTESIAN_POINT('Ctrl Pts',(0.895520212222106,-0.123823518623745,
1.45296717977858));
#6851=CARTESIAN_POINT('Ctrl Pts',(0.890059788636851,-0.101649918886749,
1.45630208793976));
#6852=CARTESIAN_POINT('Ctrl Pts',(0.886256117232622,-0.0793800000000001,
1.45861320581289));
#6853=CARTESIAN_POINT('Origin',(1.18440385848747,-0.07938,1.18440385848747));
#6854=CARTESIAN_POINT('Origin',(0.,-0.27783,0.));
#6855=CARTESIAN_POINT('',(0.404717578595295,-0.07938,1.65807299932179));
#6856=CARTESIAN_POINT('Origin',(0.,-0.07938,0.));
#6857=CARTESIAN_POINT('',(-0.404717578595296,-0.07938,1.65807299932179));
#6858=CARTESIAN_POINT('Ctrl Pts',(0.404717578595296,-0.0793800000000001,
1.65807299932179));
#6859=CARTESIAN_POINT('Ctrl Pts',(0.400393769631747,-0.101649918886749,
1.65912839404491));
#6860=CARTESIAN_POINT('Ctrl Pts',(0.394174530911058,-0.123823518623745,
1.66063136041479));
#6861=CARTESIAN_POINT('Ctrl Pts',(0.368536561654407,-0.192480977588835,
1.66658649961961));
#6862=CARTESIAN_POINT('Ctrl Pts',(0.341837165343982,-0.236152929235937,
1.67246562047521));
#6863=CARTESIAN_POINT('Ctrl Pts',(0.283214707341173,-0.303141259068211,
1.68332504372461));
#6864=CARTESIAN_POINT('Ctrl Pts',(0.244262842368623,-0.335108247315849,
1.68958170688653));
#6865=CARTESIAN_POINT('Ctrl Pts',(0.178166559972324,-0.373243761060364,
1.69769003172132));
#6866=CARTESIAN_POINT('Ctrl Pts',(0.143648558862931,-0.387888272594439,
1.70107730356824));
#6867=CARTESIAN_POINT('Ctrl Pts',(0.0717778861362652,-0.407041111792943,
1.70562212620408));
#6868=CARTESIAN_POINT('Ctrl Pts',(0.0344244045173309,-0.411552957311693,
1.706752));
#6869=CARTESIAN_POINT('Ctrl Pts',(-0.0344244045173315,-0.411552957311693,
1.706752));
#6870=CARTESIAN_POINT('Ctrl Pts',(-0.0717778861362658,-0.407041111792943,
1.70562212620408));
#6871=CARTESIAN_POINT('Ctrl Pts',(-0.143648558862932,-0.387888272594439,
1.70107730356824));
#6872=CARTESIAN_POINT('Ctrl Pts',(-0.178166559972325,-0.373243761060364,
1.69769003172132));
#6873=CARTESIAN_POINT('Ctrl Pts',(-0.244262842368624,-0.335108247315849,
1.68958170688653));
#6874=CARTESIAN_POINT('Ctrl Pts',(-0.283214707341173,-0.303141259068212,
1.68332504372461));
#6875=CARTESIAN_POINT('Ctrl Pts',(-0.341837165343982,-0.236152929235937,
1.67246562047521));
#6876=CARTESIAN_POINT('Ctrl Pts',(-0.368536561654408,-0.192480977588835,
1.66658649961961));
#6877=CARTESIAN_POINT('Ctrl Pts',(-0.394174530911059,-0.123823518623745,
1.66063136041479));
#6878=CARTESIAN_POINT('Ctrl Pts',(-0.400393769631748,-0.101649918886749,
1.65912839404491));
#6879=CARTESIAN_POINT('Ctrl Pts',(-0.404717578595297,-0.0793800000000001,
1.65807299932179));
#6880=CARTESIAN_POINT('',(-0.886256117232624,-0.07938,1.45861320581289));
#6881=CARTESIAN_POINT('Origin',(0.,-0.07938,0.));
#6882=CARTESIAN_POINT('',(-1.45861320581289,-0.07938,0.886256117232623));
#6883=CARTESIAN_POINT('Ctrl Pts',(-0.886256117232623,-0.0793800000000001,
1.45861320581289));
#6884=CARTESIAN_POINT('Ctrl Pts',(-0.890059788636852,-0.101649918886749,
1.45630208793976));
#6885=CARTESIAN_POINT('Ctrl Pts',(-0.895520212222106,-0.123823518623745,
1.45296717977858));
#6886=CARTESIAN_POINT('Ctrl Pts',(-0.917859913453974,-0.192480977588835,
1.43904931717599));
#6887=CARTESIAN_POINT('Ctrl Pts',(-0.940896403863071,-0.236152929235937,
1.4243271592157));
#6888=CARTESIAN_POINT('Ctrl Pts',(-0.990027513266105,-0.303141259068211,
1.39055359345152));
#6889=CARTESIAN_POINT('Ctrl Pts',(-1.02199477007745,-0.335108247315848,
1.36743459453896));
#6890=CARTESIAN_POINT('Ctrl Pts',(-1.07446535104584,-0.373243761060364,
1.32643091652006));
#6891=CARTESIAN_POINT('Ctrl Pts',(-1.10126842659597,-0.387888272594439,
1.30441816675528));
#6892=CARTESIAN_POINT('Ctrl Pts',(-1.15530234155453,-0.407041111792943,
1.25681160160691));
#6893=CARTESIAN_POINT('Ctrl Pts',(-1.18251418313119,-0.411552957311693,
1.23119764287622));
#6894=CARTESIAN_POINT('Ctrl Pts',(-1.23119764287622,-0.411552957311693,
1.18251418313119));
#6895=CARTESIAN_POINT('Ctrl Pts',(-1.25681160160691,-0.407041111792943,
1.15530234155453));
#6896=CARTESIAN_POINT('Ctrl Pts',(-1.30441816675528,-0.387888272594439,
1.10126842659597));
#6897=CARTESIAN_POINT('Ctrl Pts',(-1.32643091652006,-0.373243761060365,
1.07446535104584));
#6898=CARTESIAN_POINT('Ctrl Pts',(-1.36743459453896,-0.335108247315849,
1.02199477007745));
#6899=CARTESIAN_POINT('Ctrl Pts',(-1.39055359345152,-0.303141259068212,
0.990027513266106));
#6900=CARTESIAN_POINT('Ctrl Pts',(-1.4243271592157,-0.236152929235938,0.940896403863071));
#6901=CARTESIAN_POINT('Ctrl Pts',(-1.43904931717599,-0.192480977588836,
0.917859913453974));
#6902=CARTESIAN_POINT('Ctrl Pts',(-1.45296717977858,-0.123823518623746,
0.895520212222106));
#6903=CARTESIAN_POINT('Ctrl Pts',(-1.45630208793976,-0.101649918886749,
0.890059788636852));
#6904=CARTESIAN_POINT('Ctrl Pts',(-1.45861320581289,-0.0793800000000001,
0.886256117232623));
#6905=CARTESIAN_POINT('',(-1.65807299932179,-0.07938,0.404717578595295));
#6906=CARTESIAN_POINT('Origin',(0.,-0.07938,0.));
#6907=CARTESIAN_POINT('',(-1.706752,-0.411552957311693,2.08591827245526E-16));
#6908=CARTESIAN_POINT('Ctrl Pts',(-1.65807299932179,-0.0793800000000001,
0.404717578595296));
#6909=CARTESIAN_POINT('Ctrl Pts',(-1.65912839404491,-0.101649918886749,
0.400393769631747));
#6910=CARTESIAN_POINT('Ctrl Pts',(-1.66063136041479,-0.123823518623745,
0.394174530911058));
#6911=CARTESIAN_POINT('Ctrl Pts',(-1.66658649961961,-0.192480977588835,
0.368536561654407));
#6912=CARTESIAN_POINT('Ctrl Pts',(-1.67246562047521,-0.236152929235937,
0.341837165343982));
#6913=CARTESIAN_POINT('Ctrl Pts',(-1.68332504372461,-0.303141259068211,
0.283214707341173));
#6914=CARTESIAN_POINT('Ctrl Pts',(-1.68958170688653,-0.335108247315848,
0.244262842368623));
#6915=CARTESIAN_POINT('Ctrl Pts',(-1.69769003172132,-0.373243761060364,
0.178166559972324));
#6916=CARTESIAN_POINT('Ctrl Pts',(-1.70107730356824,-0.387888272594439,
0.143648558862931));
#6917=CARTESIAN_POINT('Ctrl Pts',(-1.70562212620408,-0.407041111792943,
0.0717778861362656));
#6918=CARTESIAN_POINT('Ctrl Pts',(-1.706752,-0.411552957311693,0.0344244045173313));
#6919=CARTESIAN_POINT('Ctrl Pts',(-1.706752,-0.411552957311693,2.08166817117217E-16));
#6920=CARTESIAN_POINT('',(-1.706752,-0.47628,2.09016837373834E-16));
#6921=CARTESIAN_POINT('',(-1.706752,-0.27783,2.09016837373834E-16));
#6922=CARTESIAN_POINT('Origin',(0.,-0.47628,0.));
#6923=CARTESIAN_POINT('',(-1.65807299932179,-0.07938,-0.404717578595296));
#6924=CARTESIAN_POINT('Ctrl Pts',(-1.706752,-0.411552957311693,2.0122792321331E-16));
#6925=CARTESIAN_POINT('Ctrl Pts',(-1.706752,-0.411552957311693,-0.0344244045173309));
#6926=CARTESIAN_POINT('Ctrl Pts',(-1.70562212620408,-0.407041111792943,
-0.0717778861362652));
#6927=CARTESIAN_POINT('Ctrl Pts',(-1.70107730356824,-0.387888272594439,
-0.143648558862931));
#6928=CARTESIAN_POINT('Ctrl Pts',(-1.69769003172132,-0.373243761060365,
-0.178166559972324));
#6929=CARTESIAN_POINT('Ctrl Pts',(-1.68958170688653,-0.335108247315849,
-0.244262842368623));
#6930=CARTESIAN_POINT('Ctrl Pts',(-1.68332504372461,-0.303141259068212,
-0.283214707341173));
#6931=CARTESIAN_POINT('Ctrl Pts',(-1.67246562047521,-0.236152929235938,
-0.341837165343982));
#6932=CARTESIAN_POINT('Ctrl Pts',(-1.66658649961961,-0.192480977588836,
-0.368536561654407));
#6933=CARTESIAN_POINT('Ctrl Pts',(-1.66063136041479,-0.123823518623745,
-0.394174530911059));
#6934=CARTESIAN_POINT('Ctrl Pts',(-1.65912839404491,-0.101649918886749,
-0.400393769631748));
#6935=CARTESIAN_POINT('Ctrl Pts',(-1.65807299932179,-0.0793800000000001,
-0.404717578595296));
#6936=CARTESIAN_POINT('',(-1.45861320581289,-0.07938,-0.886256117232623));
#6937=CARTESIAN_POINT('Origin',(0.,-0.07938,0.));
#6938=CARTESIAN_POINT('',(-0.886256117232623,-0.07938,-1.45861320581289));
#6939=CARTESIAN_POINT('Ctrl Pts',(-1.45861320581289,-0.0793800000000001,
-0.886256117232623));
#6940=CARTESIAN_POINT('Ctrl Pts',(-1.45630208793976,-0.101649918886749,
-0.890059788636852));
#6941=CARTESIAN_POINT('Ctrl Pts',(-1.45296717977858,-0.123823518623745,
-0.895520212222106));
#6942=CARTESIAN_POINT('Ctrl Pts',(-1.43904931717599,-0.192480977588835,
-0.917859913453974));
#6943=CARTESIAN_POINT('Ctrl Pts',(-1.4243271592157,-0.236152929235937,-0.940896403863072));
#6944=CARTESIAN_POINT('Ctrl Pts',(-1.39055359345152,-0.303141259068212,
-0.990027513266106));
#6945=CARTESIAN_POINT('Ctrl Pts',(-1.36743459453896,-0.335108247315849,
-1.02199477007745));
#6946=CARTESIAN_POINT('Ctrl Pts',(-1.32643091652006,-0.373243761060364,
-1.07446535104584));
#6947=CARTESIAN_POINT('Ctrl Pts',(-1.30441816675528,-0.387888272594439,
-1.10126842659597));
#6948=CARTESIAN_POINT('Ctrl Pts',(-1.25681160160691,-0.407041111792943,
-1.15530234155453));
#6949=CARTESIAN_POINT('Ctrl Pts',(-1.23119764287622,-0.411552957311693,
-1.18251418313119));
#6950=CARTESIAN_POINT('Ctrl Pts',(-1.18251418313119,-0.411552957311693,
-1.23119764287622));
#6951=CARTESIAN_POINT('Ctrl Pts',(-1.15530234155453,-0.407041111792943,
-1.25681160160691));
#6952=CARTESIAN_POINT('Ctrl Pts',(-1.10126842659597,-0.387888272594439,
-1.30441816675528));
#6953=CARTESIAN_POINT('Ctrl Pts',(-1.07446535104584,-0.373243761060364,
-1.32643091652006));
#6954=CARTESIAN_POINT('Ctrl Pts',(-1.02199477007745,-0.335108247315848,
-1.36743459453896));
#6955=CARTESIAN_POINT('Ctrl Pts',(-0.990027513266105,-0.303141259068211,
-1.39055359345152));
#6956=CARTESIAN_POINT('Ctrl Pts',(-0.940896403863071,-0.236152929235936,
-1.42432715921571));
#6957=CARTESIAN_POINT('Ctrl Pts',(-0.917859913453974,-0.192480977588835,
-1.43904931717599));
#6958=CARTESIAN_POINT('Ctrl Pts',(-0.895520212222106,-0.123823518623745,
-1.45296717977858));
#6959=CARTESIAN_POINT('Ctrl Pts',(-0.890059788636851,-0.101649918886749,
-1.45630208793976));
#6960=CARTESIAN_POINT('Ctrl Pts',(-0.886256117232623,-0.0793800000000001,
-1.45861320581289));
#6961=CARTESIAN_POINT('',(-0.404717578595295,-0.07938,-1.65807299932179));
#6962=CARTESIAN_POINT('Origin',(0.,-0.07938,0.));
#6963=CARTESIAN_POINT('',(0.404717578595296,-0.07938,-1.65807299932179));
#6964=CARTESIAN_POINT('Ctrl Pts',(-0.404717578595296,-0.0793800000000001,
-1.65807299932179));
#6965=CARTESIAN_POINT('Ctrl Pts',(-0.400393769631747,-0.101649918886749,
-1.65912839404491));
#6966=CARTESIAN_POINT('Ctrl Pts',(-0.394174530911058,-0.123823518623746,
-1.66063136041479));
#6967=CARTESIAN_POINT('Ctrl Pts',(-0.368536561654407,-0.192480977588836,
-1.66658649961961));
#6968=CARTESIAN_POINT('Ctrl Pts',(-0.341837165343982,-0.236152929235938,
-1.67246562047521));
#6969=CARTESIAN_POINT('Ctrl Pts',(-0.283214707341173,-0.303141259068212,
-1.68332504372461));
#6970=CARTESIAN_POINT('Ctrl Pts',(-0.244262842368623,-0.335108247315849,
-1.68958170688653));
#6971=CARTESIAN_POINT('Ctrl Pts',(-0.178166559972324,-0.373243761060364,
-1.69769003172132));
#6972=CARTESIAN_POINT('Ctrl Pts',(-0.143648558862931,-0.387888272594439,
-1.70107730356824));
#6973=CARTESIAN_POINT('Ctrl Pts',(-0.0717778861362653,-0.407041111792943,
-1.70562212620408));
#6974=CARTESIAN_POINT('Ctrl Pts',(-0.034424404517331,-0.411552957311693,
-1.706752));
#6975=CARTESIAN_POINT('Ctrl Pts',(0.0344244045173312,-0.411552957311693,
-1.706752));
#6976=CARTESIAN_POINT('Ctrl Pts',(0.0717778861362655,-0.407041111792943,
-1.70562212620408));
#6977=CARTESIAN_POINT('Ctrl Pts',(0.143648558862931,-0.387888272594439,
-1.70107730356824));
#6978=CARTESIAN_POINT('Ctrl Pts',(0.178166559972324,-0.373243761060364,
-1.69769003172132));
#6979=CARTESIAN_POINT('Ctrl Pts',(0.244262842368623,-0.335108247315849,
-1.68958170688653));
#6980=CARTESIAN_POINT('Ctrl Pts',(0.283214707341173,-0.303141259068212,
-1.68332504372461));
#6981=CARTESIAN_POINT('Ctrl Pts',(0.341837165343982,-0.236152929235937,
-1.67246562047521));
#6982=CARTESIAN_POINT('Ctrl Pts',(0.368536561654407,-0.192480977588835,
-1.66658649961961));
#6983=CARTESIAN_POINT('Ctrl Pts',(0.394174530911059,-0.123823518623745,
-1.66063136041479));
#6984=CARTESIAN_POINT('Ctrl Pts',(0.400393769631748,-0.101649918886749,
-1.65912839404491));
#6985=CARTESIAN_POINT('Ctrl Pts',(0.404717578595296,-0.0793800000000001,
-1.65807299932179));
#6986=CARTESIAN_POINT('',(0.886256117232623,-0.07938,-1.45861320581289));
#6987=CARTESIAN_POINT('Origin',(0.,-0.07938,0.));
#6988=CARTESIAN_POINT('',(1.45861320581289,-0.07938,-0.886256117232623));
#6989=CARTESIAN_POINT('Ctrl Pts',(0.886256117232623,-0.0793800000000001,
-1.45861320581289));
#6990=CARTESIAN_POINT('Ctrl Pts',(0.890059788636852,-0.101649918886749,
-1.45630208793976));
#6991=CARTESIAN_POINT('Ctrl Pts',(0.895520212222106,-0.123823518623745,
-1.45296717977858));
#6992=CARTESIAN_POINT('Ctrl Pts',(0.917859913453974,-0.192480977588835,
-1.43904931717599));
#6993=CARTESIAN_POINT('Ctrl Pts',(0.940896403863072,-0.236152929235937,
-1.4243271592157));
#6994=CARTESIAN_POINT('Ctrl Pts',(0.990027513266106,-0.303141259068211,
-1.39055359345152));
#6995=CARTESIAN_POINT('Ctrl Pts',(1.02199477007745,-0.335108247315849,-1.36743459453896));
#6996=CARTESIAN_POINT('Ctrl Pts',(1.07446535104584,-0.373243761060364,-1.32643091652006));
#6997=CARTESIAN_POINT('Ctrl Pts',(1.10126842659597,-0.387888272594439,-1.30441816675528));
#6998=CARTESIAN_POINT('Ctrl Pts',(1.15530234155453,-0.407041111792943,-1.25681160160691));
#6999=CARTESIAN_POINT('Ctrl Pts',(1.18251418313119,-0.411552957311693,-1.23119764287622));
#7000=CARTESIAN_POINT('Ctrl Pts',(1.23119764287622,-0.411552957311693,-1.18251418313119));
#7001=CARTESIAN_POINT('Ctrl Pts',(1.25681160160691,-0.407041111792943,-1.15530234155453));
#7002=CARTESIAN_POINT('Ctrl Pts',(1.30441816675528,-0.387888272594439,-1.10126842659597));
#7003=CARTESIAN_POINT('Ctrl Pts',(1.32643091652006,-0.373243761060364,-1.07446535104584));
#7004=CARTESIAN_POINT('Ctrl Pts',(1.36743459453896,-0.335108247315849,-1.02199477007745));
#7005=CARTESIAN_POINT('Ctrl Pts',(1.39055359345152,-0.303141259068212,-0.990027513266105));
#7006=CARTESIAN_POINT('Ctrl Pts',(1.4243271592157,-0.236152929235937,-0.940896403863071));
#7007=CARTESIAN_POINT('Ctrl Pts',(1.43904931717599,-0.192480977588835,-0.917859913453974));
#7008=CARTESIAN_POINT('Ctrl Pts',(1.45296717977858,-0.123823518623745,-0.895520212222106));
#7009=CARTESIAN_POINT('Ctrl Pts',(1.45630208793976,-0.101649918886749,-0.890059788636852));
#7010=CARTESIAN_POINT('Ctrl Pts',(1.45861320581289,-0.0793800000000001,
-0.886256117232623));
#7011=CARTESIAN_POINT('',(1.65807299932179,-0.07938,-0.404717578595296));
#7012=CARTESIAN_POINT('Origin',(0.,-0.07938,0.));
#7013=CARTESIAN_POINT('',(1.65807299932179,-0.07938,0.404717578595296));
#7014=CARTESIAN_POINT('Ctrl Pts',(1.65807299932179,-0.0793800000000001,
-0.404717578595296));
#7015=CARTESIAN_POINT('Ctrl Pts',(1.65912839404491,-0.101649918886749,-0.400393769631747));
#7016=CARTESIAN_POINT('Ctrl Pts',(1.66063136041479,-0.123823518623745,-0.394174530911058));
#7017=CARTESIAN_POINT('Ctrl Pts',(1.66658649961961,-0.192480977588835,-0.368536561654407));
#7018=CARTESIAN_POINT('Ctrl Pts',(1.67246562047521,-0.236152929235937,-0.341837165343982));
#7019=CARTESIAN_POINT('Ctrl Pts',(1.68332504372461,-0.303141259068212,-0.283214707341173));
#7020=CARTESIAN_POINT('Ctrl Pts',(1.68958170688653,-0.335108247315849,-0.244262842368623));
#7021=CARTESIAN_POINT('Ctrl Pts',(1.69769003172132,-0.373243761060364,-0.178166559972324));
#7022=CARTESIAN_POINT('Ctrl Pts',(1.70107730356824,-0.387888272594439,-0.143648558862931));
#7023=CARTESIAN_POINT('Ctrl Pts',(1.70562212620408,-0.407041111792943,-0.0717778861362655));
#7024=CARTESIAN_POINT('Ctrl Pts',(1.706752,-0.411552957311693,-0.0344244045173312));
#7025=CARTESIAN_POINT('Ctrl Pts',(1.706752,-0.411552957311693,0.0344244045173312));
#7026=CARTESIAN_POINT('Ctrl Pts',(1.70562212620408,-0.407041111792943,0.0717778861362655));
#7027=CARTESIAN_POINT('Ctrl Pts',(1.70107730356824,-0.387888272594439,0.143648558862931));
#7028=CARTESIAN_POINT('Ctrl Pts',(1.69769003172132,-0.373243761060364,0.178166559972324));
#7029=CARTESIAN_POINT('Ctrl Pts',(1.68958170688653,-0.335108247315849,0.244262842368623));
#7030=CARTESIAN_POINT('Ctrl Pts',(1.68332504372461,-0.303141259068212,0.283214707341173));
#7031=CARTESIAN_POINT('Ctrl Pts',(1.67246562047521,-0.236152929235937,0.341837165343982));
#7032=CARTESIAN_POINT('Ctrl Pts',(1.66658649961961,-0.192480977588835,0.368536561654407));
#7033=CARTESIAN_POINT('Ctrl Pts',(1.66063136041479,-0.123823518623745,0.394174530911058));
#7034=CARTESIAN_POINT('Ctrl Pts',(1.65912839404491,-0.101649918886749,0.400393769631747));
#7035=CARTESIAN_POINT('Ctrl Pts',(1.65807299932179,-0.0793800000000001,
0.404717578595296));
#7036=CARTESIAN_POINT('Origin',(0.,-0.07938,0.));
#7037=CARTESIAN_POINT('Origin',(0.,-0.07938,0.));
#7038=CARTESIAN_POINT('',(0.397005914195118,-0.07938,1.59456899932179));
#7039=CARTESIAN_POINT('Origin',(0.,-0.07938,0.));
#7040=CARTESIAN_POINT('Origin',(-3.33066907387547E-16,-0.07938,1.675));
#7041=CARTESIAN_POINT('Origin',(-3.33066907387547E-16,0.,1.675));
#7042=CARTESIAN_POINT('',(-0.397005914195118,-0.07938,1.59456899932179));
#7043=CARTESIAN_POINT('Ctrl Pts',(-0.397005914195119,-0.0793800000000001,
1.59456899932179));
#7044=CARTESIAN_POINT('Ctrl Pts',(-0.3886265584581,-0.123401821157026,1.59665523941937));
#7045=CARTESIAN_POINT('Ctrl Pts',(-0.373030350867485,-0.166543350814306,
1.60050712143809));
#7046=CARTESIAN_POINT('Ctrl Pts',(-0.333298652394954,-0.237231147975234,
1.60919314384089));
#7047=CARTESIAN_POINT('Ctrl Pts',(-0.311480544243687,-0.266264900654909,
1.61365775139403));
#7048=CARTESIAN_POINT('Ctrl Pts',(-0.261368388670537,-0.317195968905306,
1.62252828437015));
#7049=CARTESIAN_POINT('Ctrl Pts',(-0.233069203882014,-0.33909093068465,
1.62691869420078));
#7050=CARTESIAN_POINT('Ctrl Pts',(-0.174042761838764,-0.373586846396559,
1.63426473152765));
#7051=CARTESIAN_POINT('Ctrl Pts',(-0.14036578147155,-0.388086240756494,
1.63761964365402));
#7052=CARTESIAN_POINT('Ctrl Pts',(-0.0701778381840615,-0.407068917407805,
1.64212536811722));
#7053=CARTESIAN_POINT('Ctrl Pts',(-0.0336652739555918,-0.411552957311693,
1.643248));
#7054=CARTESIAN_POINT('Ctrl Pts',(0.0336652739555913,-0.411552957311693,
1.643248));
#7055=CARTESIAN_POINT('Ctrl Pts',(0.070177838184061,-0.407068917407805,
1.64212536811722));
#7056=CARTESIAN_POINT('Ctrl Pts',(0.140365781471549,-0.388086240756494,
1.63761964365402));
#7057=CARTESIAN_POINT('Ctrl Pts',(0.174042761838763,-0.373586846396559,
1.63426473152765));
#7058=CARTESIAN_POINT('Ctrl Pts',(0.233069203882014,-0.33909093068465,1.62691869420078));
#7059=CARTESIAN_POINT('Ctrl Pts',(0.261368388670536,-0.317195968905306,
1.62252828437015));
#7060=CARTESIAN_POINT('Ctrl Pts',(0.311480544243686,-0.266264900654908,
1.61365775139403));
#7061=CARTESIAN_POINT('Ctrl Pts',(0.333298652394954,-0.237231147975234,
1.60919314384089));
#7062=CARTESIAN_POINT('Ctrl Pts',(0.373030350867484,-0.166543350814306,
1.60050712143809));
#7063=CARTESIAN_POINT('Ctrl Pts',(0.388626558458099,-0.123401821157026,
1.59665523941937));
#7064=CARTESIAN_POINT('Ctrl Pts',(0.397005914195118,-0.07938,1.59456899932179));
#7065=CARTESIAN_POINT('Origin',(-3.33066907387547E-16,-0.07938,1.675));
#7066=CARTESIAN_POINT('Origin',(0.,-0.07938,0.));
#7067=CARTESIAN_POINT('',(-0.846804978391754,-0.07938,1.40825612658882));
#7068=CARTESIAN_POINT('Origin',(0.,-0.07938,0.));
#7069=CARTESIAN_POINT('Origin',(-1.18440385848747,-0.07938,1.18440385848747));
#7070=CARTESIAN_POINT('Origin',(-1.18440385848747,0.,1.18440385848747));
#7071=CARTESIAN_POINT('',(-1.40825612658882,-0.07938,0.846804978391753));
#7072=CARTESIAN_POINT('Ctrl Pts',(-1.40825612658882,-0.0793800000000001,
0.846804978391753));
#7073=CARTESIAN_POINT('Ctrl Pts',(-1.40380622184538,-0.123401821157026,
0.854205272175555));
#7074=CARTESIAN_POINT('Ctrl Pts',(-1.39550172959303,-0.166543350814306,
0.867957148219442));
#7075=CARTESIAN_POINT('Ctrl Pts',(-1.3735491215176,-0.237231147975235,0.902193646979983));
#7076=CARTESIAN_POINT('Ctrl Pts',(-1.36127834356734,-0.266264900654909,
0.920778333482565));
#7077=CARTESIAN_POINT('Ctrl Pts',(-1.33211611256184,-0.317195968905306,
0.962485392528369));
#7078=CARTESIAN_POINT('Ctrl Pts',(-1.31521005565926,-0.339090930684651,
0.985600426557816));
#7079=CARTESIAN_POINT('Ctrl Pts',(-1.27866649102984,-0.373586846396559,
1.03253285680459));
#7080=CARTESIAN_POINT('Ctrl Pts',(-1.25722555095714,-0.388086240756494,
1.05871835910697));
#7081=CARTESIAN_POINT('Ctrl Pts',(-1.2107812086231,-0.407068917407805,1.11153475808518));
#7082=CARTESIAN_POINT('Ctrl Pts',(-1.18575674747573,-0.411552957311693,
1.13814686046673));
#7083=CARTESIAN_POINT('Ctrl Pts',(-1.13814686046673,-0.411552957311693,
1.18575674747573));
#7084=CARTESIAN_POINT('Ctrl Pts',(-1.11153475808518,-0.407068917407805,
1.2107812086231));
#7085=CARTESIAN_POINT('Ctrl Pts',(-1.05871835910697,-0.388086240756494,
1.25722555095714));
#7086=CARTESIAN_POINT('Ctrl Pts',(-1.03253285680459,-0.373586846396559,
1.27866649102984));
#7087=CARTESIAN_POINT('Ctrl Pts',(-0.985600426557816,-0.33909093068465,
1.31521005565926));
#7088=CARTESIAN_POINT('Ctrl Pts',(-0.962485392528369,-0.317195968905306,
1.33211611256184));
#7089=CARTESIAN_POINT('Ctrl Pts',(-0.920778333482565,-0.266264900654908,
1.36127834356734));
#7090=CARTESIAN_POINT('Ctrl Pts',(-0.902193646979983,-0.237231147975234,
1.3735491215176));
#7091=CARTESIAN_POINT('Ctrl Pts',(-0.867957148219442,-0.166543350814306,
1.39550172959303));
#7092=CARTESIAN_POINT('Ctrl Pts',(-0.854205272175555,-0.123401821157026,
1.40380622184538));
#7093=CARTESIAN_POINT('Ctrl Pts',(-0.846804978391753,-0.0793800000000001,
1.40825612658882));
#7094=CARTESIAN_POINT('Origin',(-1.18440385848747,-0.07938,1.18440385848747));
#7095=CARTESIAN_POINT('Origin',(0.,-0.07938,0.));
#7096=CARTESIAN_POINT('',(-1.59456899932179,-0.07938,0.397005914195118));
#7097=CARTESIAN_POINT('Origin',(0.,-0.07938,0.));
#7098=CARTESIAN_POINT('Origin',(-1.675,-0.07938,-2.22044604925031E-16));
#7099=CARTESIAN_POINT('Origin',(-1.675,0.,-2.22044604925031E-16));
#7100=CARTESIAN_POINT('',(-1.59456899932179,-0.07938,-0.397005914195118));
#7101=CARTESIAN_POINT('',(-1.643248,-0.411552957311693,3.47540551556327E-18));
#7102=CARTESIAN_POINT('Ctrl Pts',(-1.59456899932179,-0.0793800000000001,
-0.397005914195119));
#7103=CARTESIAN_POINT('Ctrl Pts',(-1.59665523941937,-0.123401821157026,
-0.388626558458099));
#7104=CARTESIAN_POINT('Ctrl Pts',(-1.60050712143809,-0.166543350814306,
-0.373030350867485));
#7105=CARTESIAN_POINT('Ctrl Pts',(-1.60919314384089,-0.237231147975234,
-0.333298652394954));
#7106=CARTESIAN_POINT('Ctrl Pts',(-1.61365775139403,-0.266264900654909,
-0.311480544243686));
#7107=CARTESIAN_POINT('Ctrl Pts',(-1.62252828437015,-0.317195968905306,
-0.261368388670537));
#7108=CARTESIAN_POINT('Ctrl Pts',(-1.62691869420078,-0.33909093068465,-0.233069203882014));
#7109=CARTESIAN_POINT('Ctrl Pts',(-1.63426473152765,-0.373586846396559,
-0.174042761838764));
#7110=CARTESIAN_POINT('Ctrl Pts',(-1.63761964365402,-0.388086240756494,
-0.140365781471549));
#7111=CARTESIAN_POINT('Ctrl Pts',(-1.64212536811722,-0.407068917407805,
-0.0701778381840614));
#7112=CARTESIAN_POINT('Ctrl Pts',(-1.643248,-0.411552957311693,-0.0336652739555917));
#7113=CARTESIAN_POINT('Ctrl Pts',(-1.643248,-0.411552957311693,-2.0122792321331E-16));
#7114=CARTESIAN_POINT('Origin',(-1.675,-0.07938,-2.22044604925031E-16));
#7115=CARTESIAN_POINT('Ctrl Pts',(-1.643248,-0.411552957311693,-1.94289029309402E-16));
#7116=CARTESIAN_POINT('Ctrl Pts',(-1.643248,-0.411552957311693,0.0336652739555913));
#7117=CARTESIAN_POINT('Ctrl Pts',(-1.64212536811722,-0.407068917407805,
0.0701778381840609));
#7118=CARTESIAN_POINT('Ctrl Pts',(-1.63761964365402,-0.388086240756494,
0.140365781471549));
#7119=CARTESIAN_POINT('Ctrl Pts',(-1.63426473152765,-0.373586846396559,
0.174042761838763));
#7120=CARTESIAN_POINT('Ctrl Pts',(-1.62691869420078,-0.33909093068465,0.233069203882014));
#7121=CARTESIAN_POINT('Ctrl Pts',(-1.62252828437015,-0.317195968905306,
0.261368388670536));
#7122=CARTESIAN_POINT('Ctrl Pts',(-1.61365775139403,-0.266264900654909,
0.311480544243686));
#7123=CARTESIAN_POINT('Ctrl Pts',(-1.60919314384089,-0.237231147975235,
0.333298652394954));
#7124=CARTESIAN_POINT('Ctrl Pts',(-1.60050712143809,-0.166543350814306,
0.373030350867484));
#7125=CARTESIAN_POINT('Ctrl Pts',(-1.59665523941937,-0.123401821157026,
0.388626558458099));
#7126=CARTESIAN_POINT('Ctrl Pts',(-1.59456899932179,-0.0793800000000001,
0.397005914195118));
#7127=CARTESIAN_POINT('Origin',(0.,-0.07938,0.));
#7128=CARTESIAN_POINT('',(-1.40825612658882,-0.07938,-0.846804978391753));
#7129=CARTESIAN_POINT('Origin',(0.,-0.07938,0.));
#7130=CARTESIAN_POINT('Origin',(-1.18440385848747,-0.07938,-1.18440385848747));
#7131=CARTESIAN_POINT('Origin',(-1.18440385848747,0.,-1.18440385848747));
#7132=CARTESIAN_POINT('',(-0.846804978391753,-0.07938,-1.40825612658882));
#7133=CARTESIAN_POINT('Ctrl Pts',(-0.846804978391753,-0.0793800000000001,
-1.40825612658882));
#7134=CARTESIAN_POINT('Ctrl Pts',(-0.854205272175555,-0.123401821157026,
-1.40380622184538));
#7135=CARTESIAN_POINT('Ctrl Pts',(-0.867957148219442,-0.166543350814306,
-1.39550172959303));
#7136=CARTESIAN_POINT('Ctrl Pts',(-0.902193646979982,-0.237231147975234,
-1.3735491215176));
#7137=CARTESIAN_POINT('Ctrl Pts',(-0.920778333482564,-0.266264900654908,
-1.36127834356734));
#7138=CARTESIAN_POINT('Ctrl Pts',(-0.962485392528368,-0.317195968905306,
-1.33211611256184));
#7139=CARTESIAN_POINT('Ctrl Pts',(-0.985600426557816,-0.33909093068465,
-1.31521005565926));
#7140=CARTESIAN_POINT('Ctrl Pts',(-1.03253285680459,-0.373586846396559,
-1.27866649102984));
#7141=CARTESIAN_POINT('Ctrl Pts',(-1.05871835910697,-0.388086240756494,
-1.25722555095714));
#7142=CARTESIAN_POINT('Ctrl Pts',(-1.11153475808518,-0.407068917407805,
-1.2107812086231));
#7143=CARTESIAN_POINT('Ctrl Pts',(-1.13814686046673,-0.411552957311693,
-1.18575674747573));
#7144=CARTESIAN_POINT('Ctrl Pts',(-1.18575674747573,-0.411552957311693,
-1.13814686046673));
#7145=CARTESIAN_POINT('Ctrl Pts',(-1.2107812086231,-0.407068917407805,-1.11153475808518));
#7146=CARTESIAN_POINT('Ctrl Pts',(-1.25722555095714,-0.388086240756494,
-1.05871835910697));
#7147=CARTESIAN_POINT('Ctrl Pts',(-1.27866649102984,-0.373586846396559,
-1.03253285680459));
#7148=CARTESIAN_POINT('Ctrl Pts',(-1.31521005565926,-0.33909093068465,-0.985600426557816));
#7149=CARTESIAN_POINT('Ctrl Pts',(-1.33211611256184,-0.317195968905306,
-0.962485392528369));
#7150=CARTESIAN_POINT('Ctrl Pts',(-1.36127834356734,-0.266264900654909,
-0.920778333482565));
#7151=CARTESIAN_POINT('Ctrl Pts',(-1.3735491215176,-0.237231147975234,-0.902193646979983));
#7152=CARTESIAN_POINT('Ctrl Pts',(-1.39550172959303,-0.166543350814306,
-0.867957148219442));
#7153=CARTESIAN_POINT('Ctrl Pts',(-1.40380622184538,-0.123401821157026,
-0.854205272175555));
#7154=CARTESIAN_POINT('Ctrl Pts',(-1.40825612658882,-0.07938,-0.846804978391753));
#7155=CARTESIAN_POINT('Origin',(-1.18440385848747,-0.07938,-1.18440385848747));
#7156=CARTESIAN_POINT('Origin',(0.,-0.07938,0.));
#7157=CARTESIAN_POINT('',(-0.397005914195118,-0.07938,-1.59456899932179));
#7158=CARTESIAN_POINT('Origin',(0.,-0.07938,0.));
#7159=CARTESIAN_POINT('Origin',(1.11022302462516E-16,-0.07938,-1.675));
#7160=CARTESIAN_POINT('Origin',(1.11022302462516E-16,0.,-1.675));
#7161=CARTESIAN_POINT('',(0.397005914195118,-0.07938,-1.59456899932179));
#7162=CARTESIAN_POINT('Ctrl Pts',(0.397005914195119,-0.0793800000000001,
-1.59456899932179));
#7163=CARTESIAN_POINT('Ctrl Pts',(0.388626558458099,-0.123401821157026,
-1.59665523941937));
#7164=CARTESIAN_POINT('Ctrl Pts',(0.373030350867485,-0.166543350814306,
-1.60050712143809));
#7165=CARTESIAN_POINT('Ctrl Pts',(0.333298652394954,-0.237231147975234,
-1.60919314384089));
#7166=CARTESIAN_POINT('Ctrl Pts',(0.311480544243686,-0.266264900654909,
-1.61365775139403));
#7167=CARTESIAN_POINT('Ctrl Pts',(0.261368388670537,-0.317195968905306,
-1.62252828437015));
#7168=CARTESIAN_POINT('Ctrl Pts',(0.233069203882014,-0.33909093068465,-1.62691869420078));
#7169=CARTESIAN_POINT('Ctrl Pts',(0.174042761838763,-0.373586846396559,
-1.63426473152765));
#7170=CARTESIAN_POINT('Ctrl Pts',(0.140365781471549,-0.388086240756494,
-1.63761964365402));
#7171=CARTESIAN_POINT('Ctrl Pts',(0.0701778381840612,-0.407068917407805,
-1.64212536811722));
#7172=CARTESIAN_POINT('Ctrl Pts',(0.0336652739555916,-0.411552957311693,
-1.643248));
#7173=CARTESIAN_POINT('Ctrl Pts',(-0.0336652739555915,-0.411552957311693,
-1.643248));
#7174=CARTESIAN_POINT('Ctrl Pts',(-0.0701778381840612,-0.407068917407805,
-1.64212536811722));
#7175=CARTESIAN_POINT('Ctrl Pts',(-0.140365781471549,-0.388086240756494,
-1.63761964365402));
#7176=CARTESIAN_POINT('Ctrl Pts',(-0.174042761838764,-0.373586846396559,
-1.63426473152765));
#7177=CARTESIAN_POINT('Ctrl Pts',(-0.233069203882014,-0.33909093068465,
-1.62691869420078));
#7178=CARTESIAN_POINT('Ctrl Pts',(-0.261368388670536,-0.317195968905306,
-1.62252828437015));
#7179=CARTESIAN_POINT('Ctrl Pts',(-0.311480544243686,-0.266264900654908,
-1.61365775139403));
#7180=CARTESIAN_POINT('Ctrl Pts',(-0.333298652394954,-0.237231147975234,
-1.60919314384089));
#7181=CARTESIAN_POINT('Ctrl Pts',(-0.373030350867485,-0.166543350814306,
-1.60050712143809));
#7182=CARTESIAN_POINT('Ctrl Pts',(-0.388626558458099,-0.123401821157026,
-1.59665523941937));
#7183=CARTESIAN_POINT('Ctrl Pts',(-0.397005914195118,-0.07938,-1.59456899932179));
#7184=CARTESIAN_POINT('Origin',(1.11022302462516E-16,-0.07938,-1.675));
#7185=CARTESIAN_POINT('Origin',(0.,-0.07938,0.));
#7186=CARTESIAN_POINT('',(0.846804978391753,-0.07938,-1.40825612658882));
#7187=CARTESIAN_POINT('Origin',(0.,-0.07938,0.));
#7188=CARTESIAN_POINT('Origin',(1.18440385848747,-0.07938,-1.18440385848747));
#7189=CARTESIAN_POINT('Origin',(1.18440385848747,0.,-1.18440385848747));
#7190=CARTESIAN_POINT('',(1.40825612658882,-0.07938,-0.846804978391753));
#7191=CARTESIAN_POINT('Ctrl Pts',(1.40825612658882,-0.0793800000000001,
-0.846804978391753));
#7192=CARTESIAN_POINT('Ctrl Pts',(1.40380622184538,-0.123401821157026,-0.854205272175555));
#7193=CARTESIAN_POINT('Ctrl Pts',(1.39550172959303,-0.166543350814306,-0.867957148219442));
#7194=CARTESIAN_POINT('Ctrl Pts',(1.3735491215176,-0.237231147975234,-0.902193646979983));
#7195=CARTESIAN_POINT('Ctrl Pts',(1.36127834356734,-0.266264900654908,-0.920778333482565));
#7196=CARTESIAN_POINT('Ctrl Pts',(1.33211611256184,-0.317195968905306,-0.962485392528369));
#7197=CARTESIAN_POINT('Ctrl Pts',(1.31521005565926,-0.33909093068465,-0.985600426557816));
#7198=CARTESIAN_POINT('Ctrl Pts',(1.27866649102984,-0.373586846396559,-1.03253285680459));
#7199=CARTESIAN_POINT('Ctrl Pts',(1.25722555095714,-0.388086240756494,-1.05871835910697));
#7200=CARTESIAN_POINT('Ctrl Pts',(1.2107812086231,-0.407068917407805,-1.11153475808518));
#7201=CARTESIAN_POINT('Ctrl Pts',(1.18575674747573,-0.411552957311693,-1.13814686046673));
#7202=CARTESIAN_POINT('Ctrl Pts',(1.13814686046673,-0.411552957311693,-1.18575674747573));
#7203=CARTESIAN_POINT('Ctrl Pts',(1.11153475808518,-0.407068917407805,-1.2107812086231));
#7204=CARTESIAN_POINT('Ctrl Pts',(1.05871835910697,-0.388086240756494,-1.25722555095714));
#7205=CARTESIAN_POINT('Ctrl Pts',(1.03253285680459,-0.373586846396559,-1.27866649102984));
#7206=CARTESIAN_POINT('Ctrl Pts',(0.985600426557816,-0.33909093068465,-1.31521005565926));
#7207=CARTESIAN_POINT('Ctrl Pts',(0.962485392528369,-0.317195968905306,
-1.33211611256184));
#7208=CARTESIAN_POINT('Ctrl Pts',(0.920778333482565,-0.266264900654909,
-1.36127834356734));
#7209=CARTESIAN_POINT('Ctrl Pts',(0.902193646979983,-0.237231147975234,
-1.3735491215176));
#7210=CARTESIAN_POINT('Ctrl Pts',(0.867957148219442,-0.166543350814306,
-1.39550172959303));
#7211=CARTESIAN_POINT('Ctrl Pts',(0.854205272175555,-0.123401821157026,
-1.40380622184538));
#7212=CARTESIAN_POINT('Ctrl Pts',(0.846804978391753,-0.0793800000000001,
-1.40825612658882));
#7213=CARTESIAN_POINT('Origin',(1.18440385848747,-0.07938,-1.18440385848747));
#7214=CARTESIAN_POINT('Origin',(0.,-0.27783,0.));
#7215=CARTESIAN_POINT('',(-1.643248,-0.47628,2.01239840340529E-16));
#7216=CARTESIAN_POINT('Origin',(0.,-0.47628,0.));
#7217=CARTESIAN_POINT('',(-1.643248,-0.27783,2.01239840340529E-16));
#7218=CARTESIAN_POINT('',(1.59456899932179,-0.07938,0.397005914195118));
#7219=CARTESIAN_POINT('Origin',(0.,-0.07938,0.));
#7220=CARTESIAN_POINT('',(1.59456899932179,-0.07938,-0.397005914195118));
#7221=CARTESIAN_POINT('Ctrl Pts',(1.59456899932179,-0.0793800000000001,
0.397005914195118));
#7222=CARTESIAN_POINT('Ctrl Pts',(1.59665523941937,-0.123401821157026,0.388626558458099));
#7223=CARTESIAN_POINT('Ctrl Pts',(1.60050712143809,-0.166543350814306,0.373030350867485));
#7224=CARTESIAN_POINT('Ctrl Pts',(1.60919314384089,-0.237231147975234,0.333298652394954));
#7225=CARTESIAN_POINT('Ctrl Pts',(1.61365775139403,-0.266264900654909,0.311480544243686));
#7226=CARTESIAN_POINT('Ctrl Pts',(1.62252828437015,-0.317195968905306,0.261368388670537));
#7227=CARTESIAN_POINT('Ctrl Pts',(1.62691869420078,-0.33909093068465,0.233069203882014));
#7228=CARTESIAN_POINT('Ctrl Pts',(1.63426473152765,-0.373586846396559,0.174042761838764));
#7229=CARTESIAN_POINT('Ctrl Pts',(1.63761964365402,-0.388086240756494,0.140365781471549));
#7230=CARTESIAN_POINT('Ctrl Pts',(1.64212536811722,-0.407068917407805,0.0701778381840612));
#7231=CARTESIAN_POINT('Ctrl Pts',(1.643248,-0.411552957311693,0.0336652739555916));
#7232=CARTESIAN_POINT('Ctrl Pts',(1.643248,-0.411552957311693,-0.0336652739555916));
#7233=CARTESIAN_POINT('Ctrl Pts',(1.64212536811722,-0.407068917407805,-0.0701778381840612));
#7234=CARTESIAN_POINT('Ctrl Pts',(1.63761964365402,-0.388086240756494,-0.140365781471549));
#7235=CARTESIAN_POINT('Ctrl Pts',(1.63426473152765,-0.373586846396559,-0.174042761838764));
#7236=CARTESIAN_POINT('Ctrl Pts',(1.62691869420078,-0.33909093068465,-0.233069203882014));
#7237=CARTESIAN_POINT('Ctrl Pts',(1.62252828437015,-0.317195968905306,-0.261368388670537));
#7238=CARTESIAN_POINT('Ctrl Pts',(1.61365775139403,-0.266264900654909,-0.311480544243686));
#7239=CARTESIAN_POINT('Ctrl Pts',(1.60919314384089,-0.237231147975234,-0.333298652394954));
#7240=CARTESIAN_POINT('Ctrl Pts',(1.60050712143809,-0.166543350814306,-0.373030350867485));
#7241=CARTESIAN_POINT('Ctrl Pts',(1.59665523941937,-0.123401821157026,-0.388626558458099));
#7242=CARTESIAN_POINT('Ctrl Pts',(1.59456899932179,-0.07938,-0.397005914195118));
#7243=CARTESIAN_POINT('Origin',(0.,-0.07938,0.));
#7244=CARTESIAN_POINT('Origin',(0.,-0.07938,0.));
#7245=CARTESIAN_POINT('Origin',(1.675,-0.07938,0.));
#7246=CARTESIAN_POINT('Origin',(1.675,0.,0.));
#7247=CARTESIAN_POINT('Origin',(1.675,-0.07938,0.));
#7248=CARTESIAN_POINT('Origin',(0.,-0.47628,0.));
#7249=CARTESIAN_POINT('Origin',(0.,-0.07938,0.));
#7571=UNCERTAINTY_MEASURE_WITH_UNIT(LENGTH_MEASURE(0.001),#7610,
'DISTANCE_ACCURACY_VALUE',
'Maximum model space distance between geometric entities at asserted c
onnectivities');
#7579=UNCERTAINTY_MEASURE_WITH_UNIT(LENGTH_MEASURE(0.001),#7610,
'DISTANCE_ACCURACY_VALUE',
'Maximum model space distance between geometric entities at asserted c
onnectivities');
#7601=(
GEOMETRIC_REPRESENTATION_CONTEXT(3)
GLOBAL_UNCERTAINTY_ASSIGNED_CONTEXT((#7571))
GLOBAL_UNIT_ASSIGNED_CONTEXT((#7610,#7612,#7613))
REPRESENTATION_CONTEXT('','3D')
);
#7609=(
GEOMETRIC_REPRESENTATION_CONTEXT(3)
GLOBAL_UNCERTAINTY_ASSIGNED_CONTEXT((#7579))
GLOBAL_UNIT_ASSIGNED_CONTEXT((#7610,#7612,#7613))
REPRESENTATION_CONTEXT('','3D')
);
#7610=(
LENGTH_UNIT()
NAMED_UNIT(*)
SI_UNIT(.CENTI.,.METRE.)
);
#7612=(
NAMED_UNIT(*)
PLANE_ANGLE_UNIT()
SI_UNIT($,.RADIAN.)
);
#7613=(
NAMED_UNIT(*)
SI_UNIT($,.STERADIAN.)
SOLID_ANGLE_UNIT()
);
#7635=SHAPE_DEFINITION_REPRESENTATION(#7687,#7741);
#7687=PRODUCT_DEFINITION_SHAPE('',$,#7771);
#7741=SHAPE_REPRESENTATION('',(#4561),#7601);
#7749=PRODUCT_DEFINITION_CONTEXT('part definition',#7838,'design');
#7771=PRODUCT_DEFINITION('Cage','Cage',#7800,#7749);
#7800=PRODUCT_DEFINITION_FORMATION('',$,#7861);
#7838=APPLICATION_CONTEXT(
'Core Data for Automotive Mechanical Design Process');
#7839=PRODUCT_CONTEXT('part definition',#7838,'mechanical');
#7861=PRODUCT('Cage','Cage','Cage',(#7839));
#7925=COLOUR_RGB('Grey',0.48,0.52,0.57);
#7926=FILL_AREA_STYLE_COLOUR('',#7925);
#7927=FILL_AREA_STYLE('',(#7926));
#7928=SURFACE_STYLE_FILL_AREA(#7927);
#7929=SURFACE_SIDE_STYLE('',(#7928));
#7930=SURFACE_STYLE_USAGE(.BOTH.,#7929);
#7931=PRESENTATION_STYLE_ASSIGNMENT((#7930));
ENDSEC;
END-ISO-10303-21;
